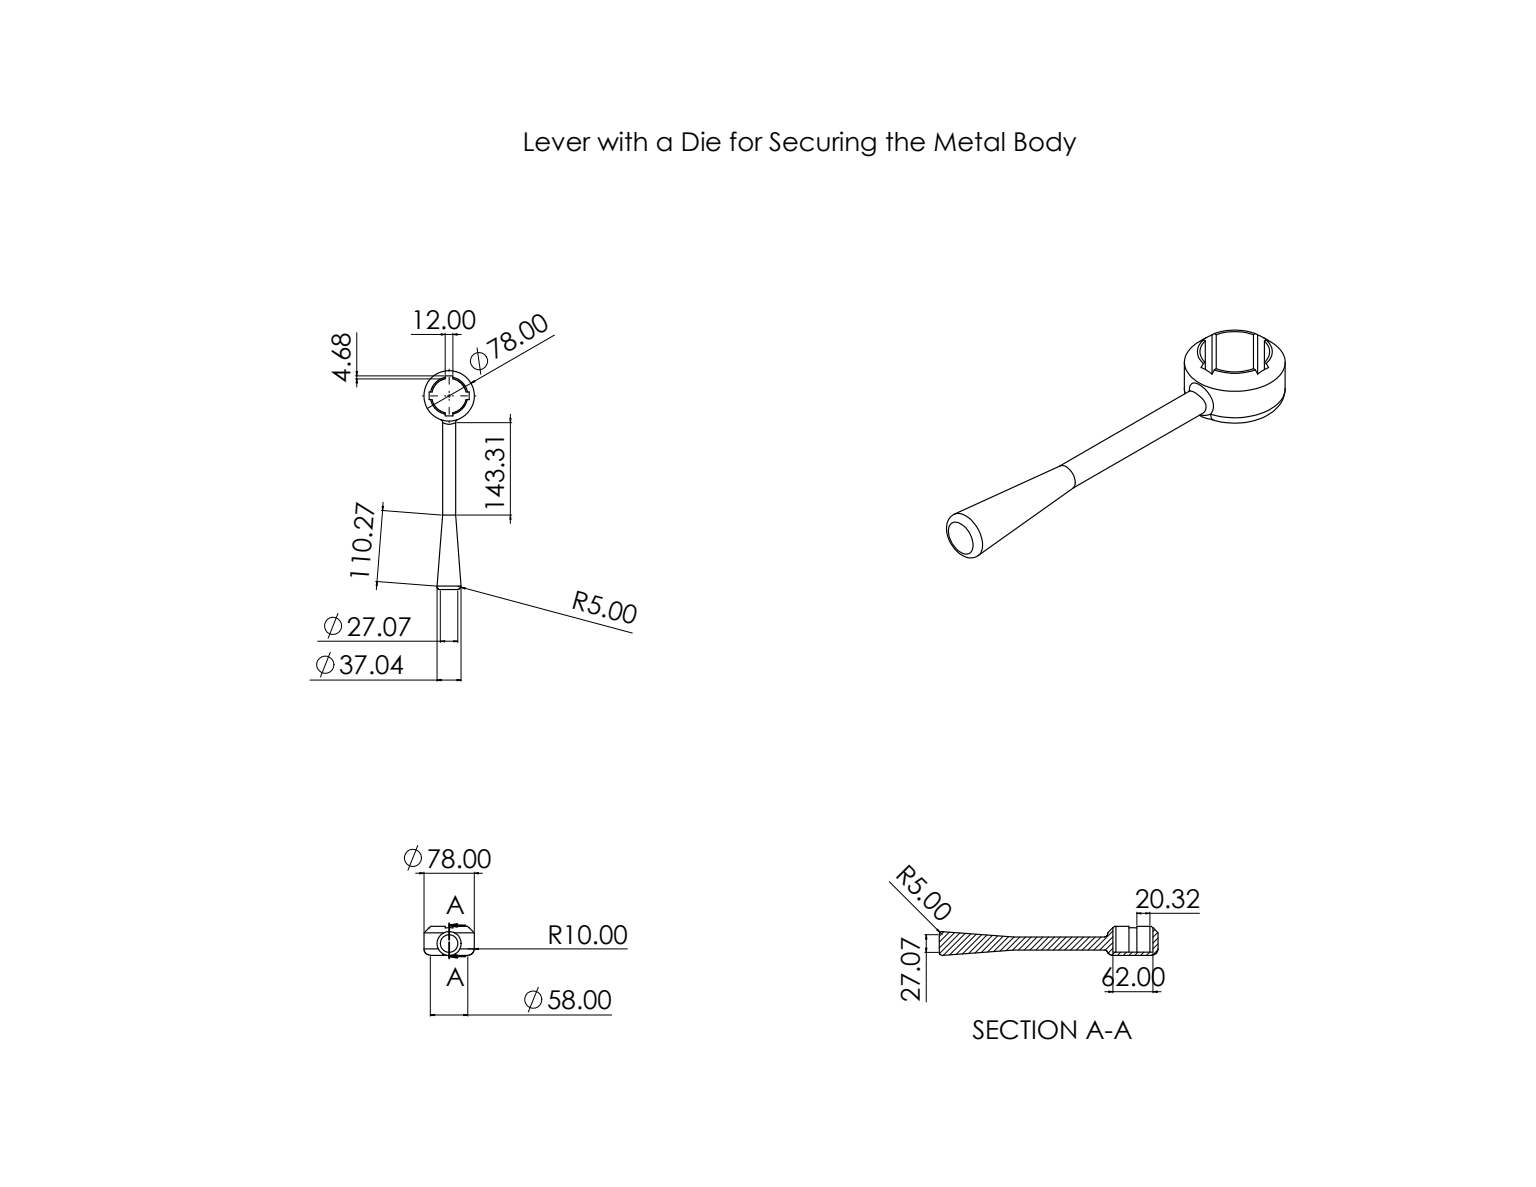
ISO-10303-21;
HEADER;
FILE_DESCRIPTION (('STEP AP214'),
    '1' );
FILE_NAME ('Lever with a Die for Securing the Metal Body.step',
    '2026-10-19T14:05:14',
    ( '' ),
    ( '' ),
    'SwSTEP 2.0',
    'SolidWorks 2025',
    '' );
FILE_SCHEMA (( 'AUTOMOTIVE_DESIGN' ));
ENDSEC;

DATA;
#5=CARTESIAN_POINT ( 'NONE',  ( 3.853297297556091738, -8.887944228554063741, 39.26446342091823993 ) ) ;
#10=CARTESIAN_POINT ( 'NONE',  ( 11.49838106938660509, -4.251877780921969219, 37.26706069643609709 ) ) ;
#13=CARTESIAN_POINT ( 'NONE',  ( 6.000000000000007994, -10.00000000000000533, 31.00000000000000711 ) ) ;
#14=CARTESIAN_POINT ( 'NONE',  ( 6.000000000000007994, 28.28385863652523824, 30.12488991936162108 ) ) ;
#20=CARTESIAN_POINT ( 'NONE',  ( -0.01963426291156584666, -6.705128248126137613, 43.99999014335539016 ) ) ;
#27=PLANE ( 'NONE',  #7404 ) ;
#29=CARTESIAN_POINT ( 'NONE',  ( -0.01628753085184865904, -6.705134819200520901, 38.99999783451422530 ) ) ;
#44=DIRECTION ( 'NONE',  ( -1.000000000000000000, 0.000000000000000000, 0.000000000000000000 ) ) ;
#54=CARTESIAN_POINT ( 'NONE',  ( 4.579605370182076030, -8.646111723837565322, 39.15306555959272572 ) ) ;
#55=CIRCLE ( 'NONE', #3026, 27.00000000000000355 ) ;
#62=CARTESIAN_POINT ( 'NONE',  ( 10.00081333311621989, 3.643253863043277363, 37.85858479645732899 ) ) ;
#67=CARTESIAN_POINT ( 'NONE',  ( -26.32489316217636954, -15.00000000000000000, 6.000000000000009770 ) ) ;
#72=CARTESIAN_POINT ( 'NONE',  ( -9.983292374582678264, 3.962892183205132479, 41.37334990339741125 ) ) ;
#82=CARTESIAN_POINT ( 'NONE',  ( -2.771370799027269349, -6.331017003992445602, 38.93346330084214202 ) ) ;
#93=EDGE_CURVE ( 'NONE', #9341, #7266, #8353, .T. ) ;
#97=CARTESIAN_POINT ( 'NONE',  ( -6.850714361783683870, -15.00000000000000000, 28.25199985127544977 ) ) ;
#112=DIRECTION ( 'NONE',  ( 0.000000000000000000, -1.000000000000000000, 0.000000000000000000 ) ) ;
#113=CARTESIAN_POINT ( 'NONE',  ( 2.825938509006990174, -14.99999999999936762, 36.77312956257851084 ) ) ;
#118=ADVANCED_FACE ( 'NONE', ( #1539 ), #6120, .T. ) ;
#122=CARTESIAN_POINT ( 'NONE',  ( 8.958048712684526294, -1.161593745032227565, 41.89873932196367434 ) ) ;
#131=CARTESIAN_POINT ( 'NONE',  ( -7.290079979600610827, 10.14749281417268811, 42.62097616879101025 ) ) ;
#134=ORIENTED_EDGE ( 'NONE', *, *, #5755, .F. ) ;
#136=ORIENTED_EDGE ( 'NONE', *, *, #3165, .T. ) ;
#157=CYLINDRICAL_SURFACE ( 'NONE', #6340, 39.00000000000002132 ) ;
#161=CARTESIAN_POINT ( 'NONE',  ( 1.729137406965966184, -11.61013223293034713, 38.97104407561932504 ) ) ;
#166=EDGE_CURVE ( 'NONE', #996, #8756, #7398, .T. ) ;
#180=ORIENTED_EDGE ( 'NONE', *, *, #6176, .F. ) ;
#181=CARTESIAN_POINT ( 'NONE',  ( -3.564217818894435563, -6.054132172044422333, 43.67637224480981217 ) ) ;
#182=DIRECTION ( 'NONE',  ( 0.000000000000000000, 0.000000000000000000, -1.000000000000000000 ) ) ;
#193=CARTESIAN_POINT ( 'NONE',  ( 5.031243191487485333, 17.19748707720165370, 38.67840086860066151 ) ) ;
#197=EDGE_CURVE ( 'NONE', #4918, #1409, #1885, .T. ) ;
#202=ORIENTED_EDGE ( 'NONE', *, *, #8489, .F. ) ;
#221=CARTESIAN_POINT ( 'NONE',  ( 0.000000000000000000, 30.00000000000000000, 0.000000000000000000 ) ) ;
#229=ORIENTED_EDGE ( 'NONE', *, *, #4215, .T. ) ;
#244=AXIS2_PLACEMENT_3D ( 'NONE', #7628, #7725, #2222 ) ;
#253=FACE_OUTER_BOUND ( 'NONE', #1428, .T. ) ;
#257=CIRCLE ( 'NONE', #6534, 9.999999999999998224 ) ;
#266=ORIENTED_EDGE ( 'NONE', *, *, #8114, .T. ) ;
#271=CARTESIAN_POINT ( 'NONE',  ( 29.24912810952613640, 29.14236109046821710, 6.000000000000000000 ) ) ;
#282=CARTESIAN_POINT ( 'NONE',  ( -9.999399707319170716, 3.681889571620033497, 37.85894501931166900 ) ) ;
#283=LINE ( 'NONE', #3269, #6859 ) ;
#285=VERTEX_POINT ( 'NONE', #824 ) ;
#292=ADVANCED_FACE ( 'NONE', ( #3127 ), #3178, .T. ) ;
#301=CARTESIAN_POINT ( 'NONE',  ( -5.022008081159694548, 11.94856982034775683, 43.35258044418206680 ) ) ;
#306=ORIENTED_EDGE ( 'NONE', *, *, #6531, .F. ) ;
#322=CARTESIAN_POINT ( 'NONE',  ( -6.860056060574510894, -3.988295739037161614, 42.78128744368499525 ) ) ;
#324=CARTESIAN_POINT ( 'NONE',  ( 3.796404955196288922E-15, 27.99999999999992184, 31.00000000000000711 ) ) ;
#328=DIRECTION ( 'NONE',  ( 8.659560562354889717E-17, -0.7071067811865512365, 0.7071067811865439090 ) ) ;
#332=CARTESIAN_POINT ( 'NONE',  ( 0.000000000000000000, 30.00000000000000000, 0.000000000000000000 ) ) ;
#351=CARTESIAN_POINT ( 'NONE',  ( 0.5362474655584705818, -6.705996766429416667, 39.00014475790622726 ) ) ;
#357=LINE ( 'NONE', #3258, #4214 ) ;
#371=CARTESIAN_POINT ( 'NONE',  ( -9.589511961634933357, 6.242300754483544267, 37.96120689204327192 ) ) ;
#386=ADVANCED_FACE ( 'NONE', ( #5330 ), #2920, .T. ) ;
#409=CARTESIAN_POINT ( 'NONE',  ( -5.034526734170375661, -14.99999999999968026, 36.79137236871326877 ) ) ;
#415=AXIS2_PLACEMENT_3D ( 'NONE', #8024, #2135, #528 ) ;
#419=AXIS2_PLACEMENT_3D ( 'NONE', #5362, #8372, #1607 ) ;
#420=CARTESIAN_POINT ( 'NONE',  ( 0.2877257019632035728, 13.29444216721321403, 38.99993006065623291 ) ) ;
#422=DIRECTION ( 'NONE',  ( 0.000000000000000000, 0.000000000000000000, -1.000000000000000000 ) ) ;
#432=CARTESIAN_POINT ( 'NONE',  ( -8.138638753224961775, -2.524951670102972834, 42.27347557256990029 ) ) ;
#434=LINE ( 'NONE', #4865, #3505 ) ;
#442=DIRECTION ( 'NONE',  ( -0.000000000000000000, 1.000000000000000000, -0.000000000000000000 ) ) ;
#443=CARTESIAN_POINT ( 'NONE',  ( 26.32489316217636954, -15.00000000000000000, -6.000000000000006217 ) ) ;
#456=ORIENTED_EDGE ( 'NONE', *, *, #4265, .F. ) ;
#458=CARTESIAN_POINT ( 'NONE',  ( -5.494756711108470526, -15.00000000000000000, 28.77837652729955309 ) ) ;
#462=CARTESIAN_POINT ( 'NONE',  ( 1.388289885975153126, 13.20576465663912735, 38.98465863473316517 ) ) ;
#466=ORIENTED_EDGE ( 'NONE', *, *, #4986, .F. ) ;
#469=B_SPLINE_CURVE_WITH_KNOTS ( 'NONE', 3,
 ( #5765, #5813, #7291, #4243, #5075, #9572, #1227, #2791, #8825, #7945, #8085, #8782, #1175, #6496, #7140, #6403, #7195, #5857, #2003, #1322, #493, #8877, #4342, #6592, #9613, #9430, #5024, #2641 ),
 .UNSPECIFIED., .F., .F.,
 ( 4, 2, 2, 2, 2, 2, 2, 2, 2, 2, 2, 2, 2, 4 ),
 ( 0.01587631186740470074, 0.01686737684520415656, 0.01785844182300361585, 0.01984057177860253096, 0.02083163675640198678, 0.02182270173420144607, 0.02281376671200090189, 0.02380483168980036118, 0.02578696164539927629, 0.02677802662319873211, 0.02776909160099819140, 0.02975122155659710305, 0.03074228653439655887, 0.03173335151219601469 ),
 .UNSPECIFIED. ) ;
#474=CARTESIAN_POINT ( 'NONE',  ( -0.4121298502407076403, 18.29573530757822653, 39.00026676411541615 ) ) ;
#483=FACE_OUTER_BOUND ( 'NONE', #5558, .T. ) ;
#484=CARTESIAN_POINT ( 'NONE',  ( 10.76768976630624763, 12.19644567871079488, 37.49298203710821298 ) ) ;
#486=CARTESIAN_POINT ( 'NONE',  ( -5.999999999999998224, -15.00000000000000000, 31.00000000000000711 ) ) ;
#487=CIRCLE ( 'NONE', #5977, 29.00000000000001776 ) ;
#493=CARTESIAN_POINT ( 'NONE',  ( 4.177119896625375972, 12.38650817078062083, 43.55397297161687220 ) ) ;
#497=CARTESIAN_POINT ( 'NONE',  ( 7.710389085651311980, -7.163490336350744059, 38.44899322361341376 ) ) ;
#503=CARTESIAN_POINT ( 'NONE',  ( -2.609644126788640328, -9.208034112191455733, 39.41000430683886435 ) ) ;
#505=CARTESIAN_POINT ( 'NONE',  ( 6.000000000000001776, 27.42469319230600533, -31.00000000000000711 ) ) ;
#507=CARTESIAN_POINT ( 'NONE',  ( 8.142856695446859305, 15.19239146806992125, 38.14742590042245496 ) ) ;
#513=ORIENTED_EDGE ( 'NONE', *, *, #7286, .F. ) ;
#519=B_SPLINE_CURVE_WITH_KNOTS ( 'NONE', 3,
 ( #6161, #3804, #5389, #1530 ),
 .UNSPECIFIED., .F., .F.,
 ( 4, 4 ),
 ( 9.813077866773594792E-18, 0.003679109433542027217 ),
 .UNSPECIFIED. ) ;
#520=CARTESIAN_POINT ( 'NONE',  ( -5.000088184532109459, 11.96127634219708291, 43.35829465038302999 ) ) ;
#521=EDGE_CURVE ( 'NONE', #3666, #5938, #5175, .T. ) ;
#528=DIRECTION ( 'NONE',  ( 0.000000000000000000, 0.000000000000000000, -1.000000000000000000 ) ) ;
#536=CARTESIAN_POINT ( 'NONE',  ( 8.924601364836032502, 14.41850173042159433, 37.96585739592215702 ) ) ;
#539=CARTESIAN_POINT ( 'NONE',  ( -28.37252191822215863, 30.00000000000000000, 6.000000000000009770 ) ) ;
#541=ADVANCED_FACE ( 'NONE', ( #6547 ), #5764, .T. ) ;
#546=EDGE_LOOP ( 'NONE', ( #4268, #589, #822, #6096, #5200 ) ) ;
#548=LINE ( 'NONE', #5078, #2613 ) ;
#549=DIRECTION ( 'NONE',  ( 0.000000000000000000, -1.000000000000000000, 0.000000000000000000 ) ) ;
#550=CARTESIAN_POINT ( 'NONE',  ( 11.07761026121386294, -5.000000000000018652, 37.39366993089406321 ) ) ;
#556=CARTESIAN_POINT ( 'NONE',  ( 0.1989820186609699559, -14.99999999999991829, 36.76396650344398864 ) ) ;
#560=CARTESIAN_POINT ( 'NONE',  ( 4.161522685292555757, 12.39367310823792145, 43.55734157098922310 ) ) ;
#569=AXIS2_PLACEMENT_3D ( 'NONE', #6747, #8347, #8246 ) ;
#570=CARTESIAN_POINT ( 'NONE',  ( -5.877770207244633838, 16.75843190384220804, 38.55650392976755114 ) ) ;
#576=CONICAL_SURFACE ( 'NONE', #6079, 10.00000000000001421, 0.07734202994352787353 ) ;
#577=VERTEX_POINT ( 'NONE', #6443 ) ;
#581=CARTESIAN_POINT ( 'NONE',  ( 0.000000000000000000, 30.00000000000000000, 0.000000000000000000 ) ) ;
#587=VECTOR ( 'NONE', #9325, 1000.000000000000000 ) ;
#589=ORIENTED_EDGE ( 'NONE', *, *, #6961, .T. ) ;
#600=FACE_OUTER_BOUND ( 'NONE', #8417, .T. ) ;
#605=CARTESIAN_POINT ( 'NONE',  ( 11.29943480391912480, 11.21459584331072712, 37.32807029000129972 ) ) ;
#610=LINE ( 'NONE', #1297, #1967 ) ;
#614=CARTESIAN_POINT ( 'NONE',  ( -10.79121869663144651, 12.07057269213421691, 37.47816149638868666 ) ) ;
#625=ORIENTED_EDGE ( 'NONE', *, *, #1724, .T. ) ;
#629=PLANE ( 'NONE',  #8412 ) ;
#640=ORIENTED_EDGE ( 'NONE', *, *, #8427, .F. ) ;
#641=CARTESIAN_POINT ( 'NONE',  ( 31.00000000000000711, -10.00000000000000533, -6.000000000000006217 ) ) ;
#642=CARTESIAN_POINT ( 'NONE',  ( 6.848559158582876449, -14.99999999999999822, 28.25275382443572525 ) ) ;
#644=AXIS2_PLACEMENT_3D ( 'NONE', #4878, #3192, #6296 ) ;
#646=EDGE_CURVE ( 'NONE', #1381, #4052, #9276, .T. ) ;
#650=CARTESIAN_POINT ( 'NONE',  ( 9.569793796949216613, 0.3522634836077675469, 37.96578825203867780 ) ) ;
#658=ORIENTED_EDGE ( 'NONE', *, *, #8055, .F. ) ;
#661=CARTESIAN_POINT ( 'NONE',  ( -6.789484220152367300, 10.67953771436871691, 38.52138918282914659 ) ) ;
#669=DIRECTION ( 'NONE',  ( 1.000000000000000000, 0.000000000000000000, 0.000000000000000000 ) ) ;
#681=CARTESIAN_POINT ( 'NONE',  ( -31.00000000000001066, 28.00044749928606791, 0.9877776005181286845 ) ) ;
#693=CARTESIAN_POINT ( 'NONE',  ( 3.829830809861694441, -15.00000000000031619, 36.77956184265733697 ) ) ;
#705=ADVANCED_FACE ( 'NONE', ( #7547 ), #776, .F. ) ;
#719=AXIS2_PLACEMENT_3D ( 'NONE', #3811, #4556, #6908 ) ;
#735=CARTESIAN_POINT ( 'NONE',  ( -6.704071815732007167, 16.26702755093696240, 38.42308545116613061 ) ) ;
#741=CARTESIAN_POINT ( 'NONE',  ( 4.138326062248817827, -15.00000000000031442, 36.78203384243531815 ) ) ;
#743=DIRECTION ( 'NONE',  ( 0.000000000000000000, 0.000000000000000000, 1.000000000000000000 ) ) ;
#750=CARTESIAN_POINT ( 'NONE',  ( 13.27537549950361750, 4.257531348894068479, 36.67105783558309895 ) ) ;
#751=ORIENTED_EDGE ( 'NONE', *, *, #8313, .F. ) ;
#755=CARTESIAN_POINT ( 'NONE',  ( -26.32489316217636954, 30.00000000000000000, 6.000000000000009770 ) ) ;
#756=EDGE_LOOP ( 'NONE', ( #6277, #2707, #2259, #1745, #813, #6889 ) ) ;
#761=EDGE_CURVE ( 'NONE', #1456, #8266, #8388, .T. ) ;
#767=CARTESIAN_POINT ( 'NONE',  ( -28.37252191822216218, 30.00000000000000000, -5.999999999999996447 ) ) ;
#776=PLANE ( 'NONE',  #7111 ) ;
#778=CARTESIAN_POINT ( 'NONE',  ( -2.813731784447083495, -15.00000000000000178, 29.91201187495168412 ) ) ;
#779=CARTESIAN_POINT ( 'NONE',  ( 8.237197373723128990, -15.00000000000000000, 27.80554943579302574 ) ) ;
#789=CARTESIAN_POINT ( 'NONE',  ( 3.173702698177182313, -14.99999999999968736, 36.77512248518149107 ) ) ;
#791=ORIENTED_EDGE ( 'NONE', *, *, #3597, .T. ) ;
#797=CARTESIAN_POINT ( 'NONE',  ( 9.984897811736454187, 3.936638391489574396, 41.37247550685020059 ) ) ;
#800=CARTESIAN_POINT ( 'NONE',  ( 6.000000000000007994, -15.00000000000000000, 31.00000000000000711 ) ) ;
#805=CARTESIAN_POINT ( 'NONE',  ( 1.221566888952841201E-22, 27.99999999999992184, -31.00000000000000711 ) ) ;
#808=CARTESIAN_POINT ( 'NONE',  ( -7.945459518470957327, -2.812008134636945655, 42.35892031214973485 ) ) ;
#811=ORIENTED_EDGE ( 'NONE', *, *, #6176, .T. ) ;
#813=ORIENTED_EDGE ( 'NONE', *, *, #5473, .F. ) ;
#814=UNCERTAINTY_MEASURE_WITH_UNIT (LENGTH_MEASURE( 1.000000000000000082E-05 ), #3122, 'distance_accuracy_value', 'NONE');
#817=CARTESIAN_POINT ( 'NONE',  ( -2.621723037464307460, -6.360998902849781089, 43.82648660254912443 ) ) ;
#822=ORIENTED_EDGE ( 'NONE', *, *, #1375, .F. ) ;
#824=CARTESIAN_POINT ( 'NONE',  ( -5.999999999999998224, -10.00000000000000533, 26.32489316217636954 ) ) ;
#825=EDGE_CURVE ( 'NONE', #7758, #8266, #9312, .T. ) ;
#843=CARTESIAN_POINT ( 'NONE',  ( 0.8530757223511000742, -15.00000000000015987, 36.76494129545336875 ) ) ;
#848=DIRECTION ( 'NONE',  ( 1.000000000000000000, 0.000000000000000000, 0.000000000000000000 ) ) ;
#851=CARTESIAN_POINT ( 'NONE',  ( 8.889207912806641687, -1.327353063715156933, 38.12328956942888425 ) ) ;
#855=DIRECTION ( 'NONE',  ( 1.000000000000000000, 0.000000000000000000, 0.000000000000000000 ) ) ;
#859=CARTESIAN_POINT ( 'NONE',  ( -9.866174171641793222, 4.958453368138042272, 41.43661138559432544 ) ) ;
#867=CARTESIAN_POINT ( 'NONE',  ( -3.062418613096201447, -11.31009261275296218, 38.88193483011423268 ) ) ;
#868=EDGE_CURVE ( 'NONE', #577, #2358, #6977, .T. ) ;
#874=VERTEX_POINT ( 'NONE', #8631 ) ;
#875=CARTESIAN_POINT ( 'NONE',  ( 3.796404955196288922E-15, 27.99999999999992184, 31.00000000000000711 ) ) ;
#888=CIRCLE ( 'NONE', #8608, 27.00000000000000355 ) ;
#897=DIRECTION ( 'NONE',  ( -0.000000000000000000, 1.000000000000000000, -0.000000000000000000 ) ) ;
#898=ORIENTED_EDGE ( 'NONE', *, *, #5824, .F. ) ;
#902=CARTESIAN_POINT ( 'NONE',  ( 6.828744152548106960, -4.017693012958108767, 42.79257513738735241 ) ) ;
#913=CARTESIAN_POINT ( 'NONE',  ( -5.512087641164731266, -8.278301759323600351, 38.98172623838953399 ) ) ;
#915=VERTEX_POINT ( 'NONE', #7983 ) ;
#916=EDGE_CURVE ( 'NONE', #5506, #2973, #8028, .T. ) ;
#917=CARTESIAN_POINT ( 'NONE',  ( -3.052805839235613661, -6.247915692633487339, 38.91814572147156781 ) ) ;
#925=CARTESIAN_POINT ( 'NONE',  ( 28.37252191822216218, 30.00000000000000000, 6.000000000000000000 ) ) ;
#926=CARTESIAN_POINT ( 'NONE',  ( 2.603483962722058287, 18.02285644508602402, 38.91836598778383660 ) ) ;
#932=EDGE_LOOP ( 'NONE', ( #6935, #6466, #9602, #8022, #6551 ) ) ;
#941=EDGE_LOOP ( 'NONE', ( #8806, #3621, #640, #6708, #7358 ) ) ;
#943=CARTESIAN_POINT ( 'NONE',  ( 0.8597079678303534145, -11.70708081913769050, 39.00058418212047684 ) ) ;
#954=CARTESIAN_POINT ( 'NONE',  ( -9.934621505046441925, 1.974978613517290427, 41.40018739529156022 ) ) ;
#960=VERTEX_POINT ( 'NONE', #7329 ) ;
#961=CARTESIAN_POINT ( 'NONE',  ( -6.703682056317219029, -9.695813972231860589, 38.42653128846041000 ) ) ;
#968=ORIENTED_EDGE ( 'NONE', *, *, #8427, .T. ) ;
#975=CARTESIAN_POINT ( 'NONE',  ( 0.7189834692050188769, -15.00000000000000000, 30.52844133725295706 ) ) ;
#985=CARTESIAN_POINT ( 'NONE',  ( -13.53485947486097984, 3.294852476641296768, 295.0000000000000000 ) ) ;
#989=CARTESIAN_POINT ( 'NONE',  ( 1.902041552336364516, -6.533359847113549890, 38.97006628291147479 ) ) ;
#992=CIRCLE ( 'NONE', #6347, 27.00000000000000355 ) ;
#993=ORIENTED_EDGE ( 'NONE', *, *, #2276, .F. ) ;
#996=VERTEX_POINT ( 'NONE', #5804 ) ;
#1009=CARTESIAN_POINT ( 'NONE',  ( -8.134414903913882000, -8.580173454344276252, 38.14378512097410123 ) ) ;
#1020=CARTESIAN_POINT ( 'NONE',  ( 10.00000000000001599, 3.294852476638864491, 41.36423575989288537 ) ) ;
#1034=CARTESIAN_POINT ( 'NONE',  ( -6.109228642973866918, 11.23818579777762139, 43.04298740074260365 ) ) ;
#1039=CARTESIAN_POINT ( 'NONE',  ( 7.734310478464688110, -8.915650141914058580, 38.22714239730741070 ) ) ;
#1041=AXIS2_PLACEMENT_3D ( 'NONE', #3721, #2820, #5974 ) ;
#1057=CARTESIAN_POINT ( 'NONE',  ( -10.00116243144523231, 2.568931457825094355, 37.85849583813012487 ) ) ;
#1064=DIRECTION ( 'NONE',  ( 0.000000000000000000, 0.000000000000000000, -1.000000000000000000 ) ) ;
#1073=EDGE_CURVE ( 'NONE', #8597, #6324, #9168, .T. ) ;
#1078=ORIENTED_EDGE ( 'NONE', *, *, #6544, .F. ) ;
#1084=LINE ( 'NONE', #8592, #6385 ) ;
#1085=CARTESIAN_POINT ( 'NONE',  ( 3.212268717265503337, -6.180893100220475667, 43.73795460093941756 ) ) ;
#1089=VERTEX_POINT ( 'NONE', #2538 ) ;
#1092=ORIENTED_EDGE ( 'NONE', *, *, #6366, .T. ) ;
#1099=ORIENTED_EDGE ( 'NONE', *, *, #6311, .T. ) ;
#1103=AXIS2_PLACEMENT_3D ( 'NONE', #3382, #9423, #7133 ) ;
#1106=CARTESIAN_POINT ( 'NONE',  ( -12.95718999772756952, -0.1032853105602432597, 36.78477091561097723 ) ) ;
#1113=ORIENTED_EDGE ( 'NONE', *, *, #9629, .F. ) ;
#1114=CARTESIAN_POINT ( 'NONE',  ( 13.53485947486097984, 3.294852476641298544, 300.0000000000000000 ) ) ;
#1116=EDGE_LOOP ( 'NONE', ( #4082, #7773, #9193 ) ) ;
#1119=DIRECTION ( 'NONE',  ( -0.000000000000000000, 1.000000000000000000, -0.000000000000000000 ) ) ;
#1141=ORIENTED_EDGE ( 'NONE', *, *, #4794, .F. ) ;
#1147=DIRECTION ( 'NONE',  ( -0.000000000000000000, 1.000000000000000000, -0.000000000000000000 ) ) ;
#1155=ORIENTED_EDGE ( 'NONE', *, *, #3946, .F. ) ;
#1156=ORIENTED_EDGE ( 'NONE', *, *, #6662, .T. ) ;
#1157=CARTESIAN_POINT ( 'NONE',  ( -9.363418156690336502, -0.2310869320007213068, 41.69859845502092099 ) ) ;
#1167=CARTESIAN_POINT ( 'NONE',  ( 0.000000000000000000, -15.00000000000000000, 0.000000000000000000 ) ) ;
#1168=CARTESIAN_POINT ( 'NONE',  ( 11.39612023638420091, -4.438368553505347869, 37.29814521415754314 ) ) ;
#1171=ADVANCED_FACE ( 'NONE', ( #3655 ), #2901, .T. ) ;
#1175=CARTESIAN_POINT ( 'NONE',  ( 7.933835403919273332, 9.390567006709300557, 42.36121793582603345 ) ) ;
#1179=CARTESIAN_POINT ( 'NONE',  ( -9.168699364306950983, 14.24186408291268435, 37.91585989658146616 ) ) ;
#1180=EDGE_CURVE ( 'NONE', #5073, #3751, #2510, .T. ) ;
#1192=CARTESIAN_POINT ( 'NONE',  ( -5.838309802342690702, -8.139381478159863903, 38.91646265135313598 ) ) ;
#1201=CARTESIAN_POINT ( 'NONE',  ( 10.56568760240365457, 12.41321854688487214, 37.54259628649076319 ) ) ;
#1203=VERTEX_POINT ( 'NONE', #2536 ) ;
#1208=EDGE_LOOP ( 'NONE', ( #6379, #6956, #7718, #4930, #229 ) ) ;
#1210=CARTESIAN_POINT ( 'NONE',  ( -9.937482190456421449, 1.998597242238694838, 41.39862281978090408 ) ) ;
#1220=DIRECTION ( 'NONE',  ( 0.000000000000000000, -0.000000000000000000, -1.000000000000000000 ) ) ;
#1221=CARTESIAN_POINT ( 'NONE',  ( 12.17954565146988699, 9.319135634659431844, 37.04959301261877869 ) ) ;
#1227=CARTESIAN_POINT ( 'NONE',  ( 9.479273386569138538, 6.546693577225376259, 41.64111890186204334 ) ) ;
#1232=CARTESIAN_POINT ( 'NONE',  ( 1.020767103194353487, -9.471900692527622567, 39.52815712443386076 ) ) ;
#1240=CARTESIAN_POINT ( 'NONE',  ( -0.8899638032320900116, -15.00000000000000000, 36.76490800571937712 ) ) ;
#1242=ORIENTED_EDGE ( 'NONE', *, *, #9562, .F. ) ;
#1243=DIRECTION ( 'NONE',  ( -1.000000000000000000, -8.673617379884034239E-17, 0.000000000000000000 ) ) ;
#1245=CARTESIAN_POINT ( 'NONE',  ( 1.332947368826647772, 13.21112352634868792, 43.95731769652755361 ) ) ;
#1255=CARTESIAN_POINT ( 'NONE',  ( -3.222268259786776667, 12.78388326438595257, 43.74320717588041418 ) ) ;
#1257=CARTESIAN_POINT ( 'NONE',  ( 4.776122516674679455E-15, -4.999999999999997335, -39.00000000000002132 ) ) ;
#1258=CARTESIAN_POINT ( 'NONE',  ( -5.999999999999998224, 30.00000000000000000, 28.37252191822216218 ) ) ;
#1262=LINE ( 'NONE', #9502, #4913 ) ;
#1266=CARTESIAN_POINT ( 'NONE',  ( 9.573718945232185362, 13.70885271580617371, 37.80730753525386945 ) ) ;
#1268=CARTESIAN_POINT ( 'NONE',  ( 0.000000000000000000, 3.294852476641296768, 184.6745183374407020 ) ) ;
#1273=DIRECTION ( 'NONE',  ( -1.000000000000000000, 0.000000000000000000, 0.000000000000000000 ) ) ;
#1287=CARTESIAN_POINT ( 'NONE',  ( -1.713217124479214482, -14.99999999999999822, 36.76766103293256549 ) ) ;
#1288=EDGE_CURVE ( 'NONE', #6115, #7606, #1262, .T. ) ;
#1292=CARTESIAN_POINT ( 'NONE',  ( 7.946841957352148711, 9.373763190100603993, 42.35574965673851722 ) ) ;
#1297=CARTESIAN_POINT ( 'NONE',  ( 10.00000000000001599, 3.294852476641296768, 300.0000000000000000 ) ) ;
#1301=CARTESIAN_POINT ( 'NONE',  ( -7.505748137593764469, 9.946373970317027968, 38.40043516335172313 ) ) ;
#1315=CARTESIAN_POINT ( 'NONE',  ( 12.79072861028647168, -0.8504798754438103181, 36.84338291468104387 ) ) ;
#1322=CARTESIAN_POINT ( 'NONE',  ( 4.473343921463067474, 12.24450654772725855, 43.48755112989530147 ) ) ;
#1331=CARTESIAN_POINT ( 'NONE',  ( -0.7293704418356496966, -15.00000000000000000, 30.52676338768143083 ) ) ;
#1338=CARTESIAN_POINT ( 'NONE',  ( 7.755618280887227378, 9.651396785365637498, 38.35455593997478729 ) ) ;
#1345=VERTEX_POINT ( 'NONE', #4379 ) ;
#1349=CARTESIAN_POINT ( 'NONE',  ( -5.501707247662611877, 11.70083553198481319, 38.70428226897013957 ) ) ;
#1360=EDGE_CURVE ( 'NONE', #3751, #9075, #4593, .T. ) ;
#1373=DIRECTION ( 'NONE',  ( -1.000000000000000000, 0.000000000000000000, 0.000000000000000000 ) ) ;
#1375=EDGE_CURVE ( 'NONE', #3666, #996, #2781, .T. ) ;
#1379=CARTESIAN_POINT ( 'NONE',  ( 0.02451486836956002016, 18.29482697815588566, 38.99999229514322252 ) ) ;
#1381=VERTEX_POINT ( 'NONE', #2170 ) ;
#1387=CARTESIAN_POINT ( 'NONE',  ( 8.139368704184242631, 9.113401726372073242, 42.27313584737455443 ) ) ;
#1396=CARTESIAN_POINT ( 'NONE',  ( -10.53299942811007917, 12.46136332956525905, 37.55180211538850443 ) ) ;
#1409=VERTEX_POINT ( 'NONE', #8914 ) ;
#1417=CARTESIAN_POINT ( 'NONE',  ( -31.00000000000000711, 27.42469319230601243, -5.999999999999996447 ) ) ;
#1418=EDGE_CURVE ( 'NONE', #1760, #8960, #8774, .T. ) ;
#1420=AXIS2_PLACEMENT_3D ( 'NONE', #332, #9364, #7235 ) ;
#1422=CARTESIAN_POINT ( 'NONE',  ( 31.00000000000001066, 28.00044749928606791, -0.9877776005181261310 ) ) ;
#1424=DIRECTION ( 'NONE',  ( 0.000000000000000000, -1.000000000000000000, 0.000000000000000000 ) ) ;
#1425=EDGE_LOOP ( 'NONE', ( #811, #2910, #8328, #5890, #5870 ) ) ;
#1427=CARTESIAN_POINT ( 'NONE',  ( 0.7189834697752452985, -15.00000000000000000, 30.52844133987663611 ) ) ;
#1428=EDGE_LOOP ( 'NONE', ( #3995, #9372, #9203, #5540, #5218, #9162, #751, #1113, #6522, #9139, #8470, #7506 ) ) ;
#1434=CARTESIAN_POINT ( 'NONE',  ( 9.994974281626689105, -6.644405053951256690, 37.70273452987021301 ) ) ;
#1442=CARTESIAN_POINT ( 'NONE',  ( -0.6382276400259029314, 13.27990715202770566, 43.99233959860035981 ) ) ;
#1446=TOROIDAL_SURFACE ( 'NONE', #4772, 13.53485947486097984, 5.000000000000000000 ) ;
#1448=CARTESIAN_POINT ( 'NONE',  ( -11.07761026121387538, -4.999999999999996447, 37.39366993089406321 ) ) ;
#1456=VERTEX_POINT ( 'NONE', #4622 ) ;
#1460=CARTESIAN_POINT ( 'NONE',  ( 28.37252191822215863, 30.00000000000000000, -6.000000000000006217 ) ) ;
#1464=VECTOR ( 'NONE', #9037, 1000.000000000000000 ) ;
#1465=CARTESIAN_POINT ( 'NONE',  ( 31.00000000000001066, 27.61361909880193011, -5.005767756411733771 ) ) ;
#1477=CARTESIAN_POINT ( 'NONE',  ( 12.57968859814066853, -1.585441976847065115, 36.91571372862268419 ) ) ;
#1484=ORIENTED_EDGE ( 'NONE', *, *, #8532, .F. ) ;
#1505=CARTESIAN_POINT ( 'NONE',  ( -0.02206928620401079830, -9.470079073673241865, 39.52734620791224529 ) ) ;
#1517=CARTESIAN_POINT ( 'NONE',  ( -1.435128562106514627, -15.00000000000000000, 30.37910620731054934 ) ) ;
#1518=DIRECTION ( 'NONE',  ( -0.000000000000000000, 1.000000000000000000, -0.000000000000000000 ) ) ;
#1520=DIRECTION ( 'NONE',  ( 0.000000000000000000, 0.000000000000000000, -1.000000000000000000 ) ) ;
#1526=CARTESIAN_POINT ( 'NONE',  ( 3.475328499451850295, -15.00000000000000000, 29.62685825611925949 ) ) ;
#1530=CARTESIAN_POINT ( 'NONE',  ( -6.000000000000005329, 30.00000000000000000, -28.37252191822215863 ) ) ;
#1532=CARTESIAN_POINT ( 'NONE',  ( 8.973048768580328627, 7.721000296853482325, 41.89150708015632318 ) ) ;
#1537=CARTESIAN_POINT ( 'NONE',  ( -26.32489316217636954, 30.00000000000000000, -5.999999999999995559 ) ) ;
#1539=FACE_OUTER_BOUND ( 'NONE', #941, .T. ) ;
#1542=DIRECTION ( 'NONE',  ( 1.000000000000000000, 0.000000000000000000, 0.000000000000000000 ) ) ;
#1545=CARTESIAN_POINT ( 'NONE',  ( -9.476145798193694958, 6.556557297351624847, 41.64275554677251989 ) ) ;
#1547=CARTESIAN_POINT ( 'NONE',  ( -1.350099534931790579, -6.635463807265971070, 43.96408345250505079 ) ) ;
#1554=ORIENTED_EDGE ( 'NONE', *, *, #7273, .T. ) ;
#1557=CARTESIAN_POINT ( 'NONE',  ( -1.781073977724889623, -11.60243029782703594, 38.96871605616770751 ) ) ;
#1575=DIRECTION ( 'NONE',  ( 1.000000000000000000, 0.000000000000000000, 0.000000000000000000 ) ) ;
#1580=CARTESIAN_POINT ( 'NONE',  ( 4.481683998297255833, -15.00000000000000000, 29.20001163310385905 ) ) ;
#1586=CARTESIAN_POINT ( 'NONE',  ( 13.12535147532733504, 5.736527869694620918, 36.72510388254905678 ) ) ;
#1596=CARTESIAN_POINT ( 'NONE',  ( -2.000890828875744099, 27.95155599451149442, -31.00000000000001066 ) ) ;
#1602=EDGE_LOOP ( 'NONE', ( #8995, #8351, #1554, #5556 ) ) ;
#1607=DIRECTION ( 'NONE',  ( -1.000000000000000000, 0.000000000000000000, 0.000000000000000000 ) ) ;
#1614=CARTESIAN_POINT ( 'NONE',  ( 6.611979057083408939, -4.234811449640147885, 42.87340679459065029 ) ) ;
#1617=LINE ( 'NONE', #3033, #2215 ) ;
#1626=CARTESIAN_POINT ( 'NONE',  ( 8.821391692846543009, -15.00000000000000178, 36.98463040684644909 ) ) ;
#1632=CARTESIAN_POINT ( 'NONE',  ( 8.719889270409380444, -1.642155660953823926, 38.16040262559969420 ) ) ;
#1635=LINE ( 'NONE', #7567, #2917 ) ;
#1647=CARTESIAN_POINT ( 'NONE',  ( -1.109536816265070058, -6.661247609618464516, 38.99263510515930165 ) ) ;
#1657=AXIS2_PLACEMENT_3D ( 'NONE', #3222, #3024, #3978 ) ;
#1659=CARTESIAN_POINT ( 'NONE',  ( 8.955614711045242871, -1.166416508362459137, 41.89990723123212035 ) ) ;
#1661=CARTESIAN_POINT ( 'NONE',  ( 31.00000000000000711, 27.42469319230600533, -6.000000000000006217 ) ) ;
#1662=DIRECTION ( 'NONE',  ( 0.000000000000000000, -0.000000000000000000, -1.000000000000000000 ) ) ;
#1664=CARTESIAN_POINT ( 'NONE',  ( -26.32489316217636954, -10.00000000000000533, 6.000000000000009770 ) ) ;
#1671=CIRCLE ( 'NONE', #7981, 18.51991245392837371 ) ;
#1685=CARTESIAN_POINT ( 'NONE',  ( 3.009843071917527535, -11.32397619240443376, 38.88603724746761969 ) ) ;
#1688=CARTESIAN_POINT ( 'NONE',  ( 10.00000000000001421, 3.294852476641296768, 184.6745183374407020 ) ) ;
#1689=DIRECTION ( 'NONE',  ( -0.000000000000000000, 1.000000000000000000, -0.000000000000000000 ) ) ;
#1718=VERTEX_POINT ( 'NONE', #1537 ) ;
#1719=DIRECTION ( 'NONE',  ( 0.000000000000000000, 0.000000000000000000, -1.000000000000000000 ) ) ;
#1723=DIRECTION ( 'NONE',  ( 0.000000000000000000, 0.000000000000000000, 1.000000000000000000 ) ) ;
#1724=EDGE_CURVE ( 'NONE', #6115, #7120, #1635, .T. ) ;
#1737=VECTOR ( 'NONE', #6997, 1000.000000000000000 ) ;
#1739=CARTESIAN_POINT ( 'NONE',  ( -0.6917606027332897645, -6.703808575055850483, 43.99931531168492427 ) ) ;
#1745=ORIENTED_EDGE ( 'NONE', *, *, #646, .F. ) ;
#1747=CARTESIAN_POINT ( 'NONE',  ( -13.29481821656429652, 3.809926294481188691, 36.66398517656647016 ) ) ;
#1755=DIRECTION ( 'NONE',  ( 0.000000000000000000, 0.000000000000000000, -1.000000000000000000 ) ) ;
#1760=VERTEX_POINT ( 'NONE', #8201 ) ;
#1769=CARTESIAN_POINT ( 'NONE',  ( 5.817259163329850935, -4.845482602429197705, 43.12805808941161700 ) ) ;
#1785=DIRECTION ( 'NONE',  ( -1.000000000000000000, 0.000000000000000000, 0.000000000000000000 ) ) ;
#1792=EDGE_CURVE ( 'NONE', #8477, #9075, #4610, .T. ) ;
#1793=CARTESIAN_POINT ( 'NONE',  ( -13.18364556721897429, 5.298907180833983155, 36.70413758096341184 ) ) ;
#1798=CARTESIAN_POINT ( 'NONE',  ( 0.000000000000000000, -15.00000000000000000, 0.000000000000000000 ) ) ;
#1821=CARTESIAN_POINT ( 'NONE',  ( -0.6444271763597331226, 13.27961199780309798, 43.99218798305987121 ) ) ;
#1826=CARTESIAN_POINT ( 'NONE',  ( -0.01628753085184865904, -6.705134819200520901, 38.99999783451422530 ) ) ;
#1828=VERTEX_POINT ( 'NONE', #13 ) ;
#1831=CARTESIAN_POINT ( 'NONE',  ( 2.000890828875750316, 27.95155599451150152, 31.00000000000001421 ) ) ;
#1836=CARTESIAN_POINT ( 'NONE',  ( 0.000000000000000000, 19.99999999999982236, 39.00000000000002132 ) ) ;
#1845=CARTESIAN_POINT ( 'NONE',  ( -6.066055860285464618, -4.695835677951882836, 38.62830766617436495 ) ) ;
#1856=DIRECTION ( 'NONE',  ( 0.000000000000000000, 0.000000000000000000, 1.000000000000000000 ) ) ;
#1865=CARTESIAN_POINT ( 'NONE',  ( -13.15180771621593792, 5.587517427209601095, 36.71572060651241287 ) ) ;
#1870=ORIENTED_EDGE ( 'NONE', *, *, #3165, .F. ) ;
#1874=DIRECTION ( 'NONE',  ( 1.000000000000000000, 0.000000000000000000, 0.000000000000000000 ) ) ;
#1885=CIRCLE ( 'NONE', #8359, 27.00000000000000355 ) ;
#1887=ORIENTED_EDGE ( 'NONE', *, *, #7554, .F. ) ;
#1888=CARTESIAN_POINT ( 'NONE',  ( -9.211085773935334231, -0.6384518674459094267, 38.05061636510622236 ) ) ;
#1901=CARTESIAN_POINT ( 'NONE',  ( 8.239768008128093513, 15.08660039710901657, 38.12250742654718039 ) ) ;
#1914=CARTESIAN_POINT ( 'NONE',  ( -12.77877500440332170, 7.486973052590117028, 36.84754185667136994 ) ) ;
#1921=CARTESIAN_POINT ( 'NONE',  ( -8.124805145827266983, -15.00000000000000000, 36.91741529765116780 ) ) ;
#1923=VERTEX_POINT ( 'NONE', #8594 ) ;
#1928=CARTESIAN_POINT ( 'NONE',  ( 6.697485916193928190, 16.26204223369385460, 38.42259331311452542 ) ) ;
#1936=CARTESIAN_POINT ( 'NONE',  ( -8.755997409701210543, -1.617811598344234048, 38.15348978656172818 ) ) ;
#1945=CARTESIAN_POINT ( 'NONE',  ( -29.24912810952613640, 29.14236109046821710, -5.999999999999996447 ) ) ;
#1946=CARTESIAN_POINT ( 'NONE',  ( 7.754649722547835466, 15.49890469874339871, 38.22487108103376841 ) ) ;
#1967=VECTOR ( 'NONE', #9594, 1000.000000000000000 ) ;
#1971=CARTESIAN_POINT ( 'NONE',  ( -8.643728504328578310, -6.580413251913810768, 38.16276976896127593 ) ) ;
#1973=CARTESIAN_POINT ( 'NONE',  ( 13.53485947486097984, 3.294852476641298544, 295.0000000000000000 ) ) ;
#1979=CARTESIAN_POINT ( 'NONE',  ( 7.068581912135081247, 16.00861037931602127, 38.35581056696806712 ) ) ;
#1985=EDGE_LOOP ( 'NONE', ( #6670, #9493, #5390, #2665, #2718 ) ) ;
#1987=CARTESIAN_POINT ( 'NONE',  ( -8.768074816142425121, 14.61274975128556264, 38.00682554133690871 ) ) ;
#2003=CARTESIAN_POINT ( 'NONE',  ( 5.048957243282207408, 11.93285829901166295, 43.34552440119345107 ) ) ;
#2010=CYLINDRICAL_SURFACE ( 'NONE', #8911, 27.00000000000000355 ) ;
#2013=CARTESIAN_POINT ( 'NONE',  ( -11.07761026121418091, -4.999999999999992006, 37.39366993089505797 ) ) ;
#2016=ADVANCED_FACE ( 'NONE', ( #9583 ), #2010, .F. ) ;
#2020=CARTESIAN_POINT ( 'NONE',  ( 0.5600451362621369222, 13.28348936595889107, 38.99807195037084995 ) ) ;
#2039=CYLINDRICAL_SURFACE ( 'NONE', #8669, 39.00000000000002132 ) ;
#2047=DIRECTION ( 'NONE',  ( -0.000000000000000000, 0.000000000000000000, -1.000000000000000000 ) ) ;
#2054=LINE ( 'NONE', #5774, #6969 ) ;
#2060=CARTESIAN_POINT ( 'NONE',  ( -8.237197373723452287, -14.99999999999999822, 27.80554943579402405 ) ) ;
#2066=CARTESIAN_POINT ( 'NONE',  ( 6.124541788014690624, 11.22654513750760330, 43.03812152903055477 ) ) ;
#2077=CARTESIAN_POINT ( 'NONE',  ( -8.102752655081463473, 15.22736282390319040, 38.15602848768372723 ) ) ;
#2085=ORIENTED_EDGE ( 'NONE', *, *, #1360, .T. ) ;
#2086=CARTESIAN_POINT ( 'NONE',  ( 6.000000000000001776, 30.00000000000000000, -31.00000000000000711 ) ) ;
#2088=CARTESIAN_POINT ( 'NONE',  ( 0.000000000000000000, 3.294852476641296768, 300.0000000000000000 ) ) ;
#2091=CARTESIAN_POINT ( 'NONE',  ( -5.999999999999998224, -10.00000000000000533, 31.00000000000000711 ) ) ;
#2098=CARTESIAN_POINT ( 'NONE',  ( 6.439978105601112524E-15, 18.29485247664131009, 39.00000000000002132 ) ) ;
#2104=CARTESIAN_POINT ( 'NONE',  ( -2.470322857848779918, -15.00000000000000000, 30.03203418347360909 ) ) ;
#2112=CARTESIAN_POINT ( 'NONE',  ( 5.928038920598607042, 16.73037627209208367, 38.54880476822177116 ) ) ;
#2123=EDGE_LOOP ( 'NONE', ( #8637, #6822, #6319, #1242, #7196 ) ) ;
#2125=CARTESIAN_POINT ( 'NONE',  ( -6.594791314557400419, 10.84011732630675695, 42.87949548222016460 ) ) ;
#2130=EDGE_CURVE ( 'NONE', #3412, #3666, #7250, .T. ) ;
#2135=DIRECTION ( 'NONE',  ( 0.000000000000000000, -1.000000000000000000, 0.000000000000000000 ) ) ;
#2136=ORIENTED_EDGE ( 'NONE', *, *, #9140, .F. ) ;
#2154=CARTESIAN_POINT ( 'NONE',  ( 0.4198266780023428568, -14.99999999999984190, 36.76416815479328903 ) ) ;
#2156=DIRECTION ( 'NONE',  ( -1.224646799147353207E-16, 1.000000000000000000, 0.000000000000000000 ) ) ;
#2157=LINE ( 'NONE', #2954, #6691 ) ;
#2158=CARTESIAN_POINT ( 'NONE',  ( 9.981004741123138402, 4.018542934133168210, 37.86365196549936485 ) ) ;
#2159=ORIENTED_EDGE ( 'NONE', *, *, #8489, .T. ) ;
#2166=CARTESIAN_POINT ( 'NONE',  ( -8.731905042198331302, 8.252142515900809272, 38.15876855944379287 ) ) ;
#2170=CARTESIAN_POINT ( 'NONE',  ( -0.01963426291156584666, -6.705128248126137613, 43.99999014335539016 ) ) ;
#2172=ORIENTED_EDGE ( 'NONE', *, *, #3907, .F. ) ;
#2182=CARTESIAN_POINT ( 'NONE',  ( 0.6536441304786463347, -6.706450183173051194, 44.00066613171647845 ) ) ;
#2186=CARTESIAN_POINT ( 'NONE',  ( 4.007921376381021084, 27.80323177039520033, -31.00000000000000711 ) ) ;
#2188=LINE ( 'NONE', #6792, #4017 ) ;
#2189=CARTESIAN_POINT ( 'NONE',  ( 31.00000000000000355, 27.99909559099847911, 2.017392264862529760 ) ) ;
#2193=FACE_OUTER_BOUND ( 'NONE', #5768, .T. ) ;
#2196=( GEOMETRIC_REPRESENTATION_CONTEXT ( 3 ) GLOBAL_UNCERTAINTY_ASSIGNED_CONTEXT ( ( #3771 ) ) GLOBAL_UNIT_ASSIGNED_CONTEXT ( ( #4528, #4383, #2880 ) ) REPRESENTATION_CONTEXT ( 'NONE', 'WORKASPACE' ) );
#2201=CARTESIAN_POINT ( 'NONE',  ( 9.350174078884196049, -0.2661211825927956576, 41.70529496454247464 ) ) ;
#2211=CARTESIAN_POINT ( 'NONE',  ( -4.149849522310169903, 12.39897866860190767, 43.55983959218083612 ) ) ;
#2215=VECTOR ( 'NONE', #2887, 1000.000000000000000 ) ;
#2220=CARTESIAN_POINT ( 'NONE',  ( 6.000000000000001776, 28.28385863652523824, -30.12488991936162108 ) ) ;
#2222=DIRECTION ( 'NONE',  ( 0.001963426291157480824, 0.9999980724767419948, 0.000000000000000000 ) ) ;
#2223=AXIS2_PLACEMENT_3D ( 'NONE', #5491, #3350, #1723 ) ;
#2234=CARTESIAN_POINT ( 'NONE',  ( -10.00000000000001599, 3.294852476641298100, 300.0000000000000000 ) ) ;
#2243=CARTESIAN_POINT ( 'NONE',  ( 0.000000000000000000, -15.00000000000000000, 0.000000000000000000 ) ) ;
#2246=CARTESIAN_POINT ( 'NONE',  ( 0.4484383372385683519, -15.00000000000000000, 30.56042761519584872 ) ) ;
#2250=CARTESIAN_POINT ( 'NONE',  ( 26.32489316217636954, -15.00000000000000000, 6.000000000000000000 ) ) ;
#2256=CARTESIAN_POINT ( 'NONE',  ( 12.43148144571613223, -2.046608012193396942, 36.96605690027389102 ) ) ;
#2259=ORIENTED_EDGE ( 'NONE', *, *, #2546, .F. ) ;
#2260=CARTESIAN_POINT ( 'NONE',  ( -26.32489316217636954, -15.00000000000000000, 6.000000000000009770 ) ) ;
#2265=DIRECTION ( 'NONE',  ( -0.000000000000000000, -0.000000000000000000, 1.000000000000000000 ) ) ;
#2268=CARTESIAN_POINT ( 'NONE',  ( -1.306712379120655632, 13.21469178175683190, 43.95913021330854065 ) ) ;
#2276=EDGE_CURVE ( 'NONE', #2374, #915, #7159, .T. ) ;
#2280=DIRECTION ( 'NONE',  ( 0.000000000000000000, -1.000000000000000000, 0.000000000000000000 ) ) ;
#2281=CARTESIAN_POINT ( 'NONE',  ( -0.02610464500743471528, -11.70511861050984947, 38.99999126342864741 ) ) ;
#2283=CARTESIAN_POINT ( 'NONE',  ( 5.000171879512024908, -8.491196122513333222, 39.08124479469799439 ) ) ;
#2298=VERTEX_POINT ( 'NONE', #5332 ) ;
#2303=FACE_OUTER_BOUND ( 'NONE', #5668, .T. ) ;
#2306=CARTESIAN_POINT ( 'NONE',  ( 6.332203200428770273, -7.897660556950563127, 38.80169624000574657 ) ) ;
#2310=EDGE_LOOP ( 'NONE', ( #7054, #6754 ) ) ;
#2311=CARTESIAN_POINT ( 'NONE',  ( 9.194894985997349224, -0.6766425519222662999, 38.05435396104630996 ) ) ;
#2314=ADVANCED_FACE ( 'NONE', ( #2303 ), #8291, .T. ) ;
#2322=CARTESIAN_POINT ( 'NONE',  ( -2.620222824297394393, 12.96846514759271152, 43.83512211430772965 ) ) ;
#2323=B_SPLINE_CURVE_WITH_KNOTS ( 'NONE', 3,
 ( #8977, #6686, #9721, #1460 ),
 .UNSPECIFIED., .F., .F.,
 ( 4, 4 ),
 ( 9.813077866773594792E-18, 0.003679109433542027217 ),
 .UNSPECIFIED. ) ;
#2325=CARTESIAN_POINT ( 'NONE',  ( -9.351925007598564932, -0.2614073996901185026, 41.70440666569142252 ) ) ;
#2330=VERTEX_POINT ( 'NONE', #5229 ) ;
#2334=CARTESIAN_POINT ( 'NONE',  ( 6.000000000000007994, 30.00000000000000000, 26.32489316217636954 ) ) ;
#2337=DIRECTION ( 'NONE',  ( -1.000000000000000000, 0.000000000000000000, 0.000000000000000000 ) ) ;
#2341=LINE ( 'NONE', #2234, #8706 ) ;
#2349=AXIS2_PLACEMENT_3D ( 'NONE', #7819, #1785, #7766 ) ;
#2353=CARTESIAN_POINT ( 'NONE',  ( 8.119362783942410289, -15.00000000000000000, 36.91696022903513352 ) ) ;
#2358=VERTEX_POINT ( 'NONE', #3994 ) ;
#2362=DIRECTION ( 'NONE',  ( -0.000000000000000000, 0.000000000000000000, -1.000000000000000000 ) ) ;
#2363=CARTESIAN_POINT ( 'NONE',  ( 6.000000000000007994, 30.00000000000000000, 28.37252191822215863 ) ) ;
#2365=CARTESIAN_POINT ( 'NONE',  ( -0.02206928620401079830, -9.470079073673241865, 39.52734620791224529 ) ) ;
#2366=VECTOR ( 'NONE', #44, 1000.000000000000000 ) ;
#2370=DIRECTION ( 'NONE',  ( 0.000000000000000000, 0.000000000000000000, -1.000000000000000000 ) ) ;
#2374=VERTEX_POINT ( 'NONE', #7793 ) ;
#2377=ORIENTED_EDGE ( 'NONE', *, *, #5999, .T. ) ;
#2383=ADVANCED_FACE ( 'NONE', ( #4787 ), #8533, .F. ) ;
#2389=ORIENTED_EDGE ( 'NONE', *, *, #4010, .F. ) ;
#2398=CIRCLE ( 'NONE', #5866, 5.000000000000004441 ) ;
#2409=CARTESIAN_POINT ( 'NONE',  ( 3.017393985291145331, -6.258907930525880126, 38.92018111626612864 ) ) ;
#2426=CARTESIAN_POINT ( 'NONE',  ( -3.886469093799143071, -5.959786720418388306, 38.86437971944521053 ) ) ;
#2436=ORIENTED_EDGE ( 'NONE', *, *, #2546, .T. ) ;
#2453=DIRECTION ( 'NONE',  ( 0.000000000000000000, 0.000000000000000000, -1.000000000000000000 ) ) ;
#2460=LINE ( 'NONE', #5494, #1737 ) ;
#2464=LINE ( 'NONE', #5498, #2936 ) ;
#2467=CARTESIAN_POINT ( 'NONE',  ( -3.270419483466965982, -6.161042622928358803, 43.72827664804632519 ) ) ;
#2474=CARTESIAN_POINT ( 'NONE',  ( -7.065584702402819772, -3.825344972707461100, 38.47648702749351912 ) ) ;
#2483=CARTESIAN_POINT ( 'NONE',  ( -31.00000000000000711, -10.00000000000000533, 6.000000000000009770 ) ) ;
#2489=DIRECTION ( 'NONE',  ( 0.000000000000000000, -1.000000000000000000, 0.000000000000000000 ) ) ;
#2494=ORIENTED_EDGE ( 'NONE', *, *, #8267, .T. ) ;
#2498=AXIS2_PLACEMENT_3D ( 'NONE', #67, #2362, #5396 ) ;
#2499=CARTESIAN_POINT ( 'NONE',  ( 4.404177573089986808, -5.731393103011397372, 38.82088277608229276 ) ) ;
#2508=CARTESIAN_POINT ( 'NONE',  ( 31.00000000000000711, 27.42469319230601243, 6.000000000000000000 ) ) ;
#2510=LINE ( 'NONE', #4069, #5366 ) ;
#2518=CARTESIAN_POINT ( 'NONE',  ( -9.982669663254970516, 3.970470032139787442, 41.37368756539773074 ) ) ;
#2536=CARTESIAN_POINT ( 'NONE',  ( 28.37252191822215863, 30.00000000000000000, -6.000000000000006217 ) ) ;
#2538=CARTESIAN_POINT ( 'NONE',  ( -13.53485947486097984, 3.294852476641296768, 300.0000000000000000 ) ) ;
#2544=CARTESIAN_POINT ( 'NONE',  ( -9.916130411093226016, 4.630053343978718594, 41.40967485888758404 ) ) ;
#2546=EDGE_CURVE ( 'NONE', #4052, #6324, #469, .T. ) ;
#2550=CARTESIAN_POINT ( 'NONE',  ( 6.030565054738658226, -4.722726170226616560, 38.63317537858744544 ) ) ;
#2571=CARTESIAN_POINT ( 'NONE',  ( -10.01570558914089126, -6.581988155506046212, 37.69304774390490564 ) ) ;
#2575=APPLICATION_CONTEXT ( 'automotive_design' ) ;
#2579=DIRECTION ( 'NONE',  ( 0.000000000000000000, 0.000000000000000000, -1.000000000000000000 ) ) ;
#2583=CARTESIAN_POINT ( 'NONE',  ( 12.93945410785518924, -0.2138153430966752699, 36.79108894230666493 ) ) ;
#2586=FACE_OUTER_BOUND ( 'NONE', #3346, .T. ) ;
#2588=AXIS2_PLACEMENT_3D ( 'NONE', #1268, #5711, #6396 ) ;
#2597=CARTESIAN_POINT ( 'NONE',  ( -6.000000000000005329, -15.00000000000000000, -31.00000000000000711 ) ) ;
#2600=CARTESIAN_POINT ( 'NONE',  ( -13.23256407018424063, 1.700849823644902115, 36.68651977394890196 ) ) ;
#2613=VECTOR ( 'NONE', #3594, 1000.000000000000000 ) ;
#2618=VECTOR ( 'NONE', #1518, 1000.000000000000000 ) ;
#2628=CARTESIAN_POINT ( 'NONE',  ( -12.85843207060513116, 7.233932487497670927, 36.81975545894231061 ) ) ;
#2636=PLANE ( 'NONE',  #2823 ) ;
#2641=CARTESIAN_POINT ( 'NONE',  ( 0.01843853345419280837, 13.29483547765106799, 43.99999130734108377 ) ) ;
#2643=CARTESIAN_POINT ( 'NONE',  ( 0.000000000000000000, 19.99999999999982236, -39.00000000000002132 ) ) ;
#2659=CARTESIAN_POINT ( 'NONE',  ( 0.01843853345419369655, 13.29483547765106977, 43.99999130734107666 ) ) ;
#2665=ORIENTED_EDGE ( 'NONE', *, *, #2977, .T. ) ;
#2669=CARTESIAN_POINT ( 'NONE',  ( -7.944109461005667505, -2.787611319100306240, 42.35690170190217430 ) ) ;
#2676=ORIENTED_EDGE ( 'NONE', *, *, #4215, .F. ) ;
#2704=CARTESIAN_POINT ( 'NONE',  ( 0.01225733702461903260, 18.29484822699931001, 38.99999871588790512 ) ) ;
#2705=CARTESIAN_POINT ( 'NONE',  ( -10.07733521876669336, -14.99999999999807621, 37.15918820280854362 ) ) ;
#2707=ORIENTED_EDGE ( 'NONE', *, *, #1073, .T. ) ;
#2711=CONICAL_SURFACE ( 'NONE', #7777, 39.00000000000002132, 0.7853981633974431720 ) ;
#2712=CARTESIAN_POINT ( 'NONE',  ( 3.604595221023451312, 12.64709689291967187, 38.88259557046998083 ) ) ;
#2718=ORIENTED_EDGE ( 'NONE', *, *, #9262, .T. ) ;
#2720=CARTESIAN_POINT ( 'NONE',  ( 0.02451486836953505749, 18.29482697815588921, 38.99999229514322252 ) ) ;
#2722=DIRECTION ( 'NONE',  ( 1.776356839400250465E-15, 0.000000000000000000, -1.000000000000000000 ) ) ;
#2748=CARTESIAN_POINT ( 'NONE',  ( 0.000000000000000000, 30.00000000000000000, 0.000000000000000000 ) ) ;
#2751=CARTESIAN_POINT ( 'NONE',  ( 10.23650415797109758, -5.544651734979271218, 37.65358413834264439 ) ) ;
#2758=CARTESIAN_POINT ( 'NONE',  ( 0.08302437902281271931, -15.00000000000000000, 30.58222658736175248 ) ) ;
#2759=ORIENTED_EDGE ( 'NONE', *, *, #2130, .F. ) ;
#2766=CARTESIAN_POINT ( 'NONE',  ( 4.330416360834490774, 17.51076624374514523, 38.76727366216590553 ) ) ;
#2771=PRODUCT_DEFINITION_CONTEXT ( 'detailed design', #2575, 'design' ) ;
#2777=CARTESIAN_POINT ( 'NONE',  ( -0.3099780140802378403, 13.29544103063097893, 44.00030096464039531 ) ) ;
#2781=LINE ( 'NONE', #5801, #8763 ) ;
#2785=DIRECTION ( 'NONE',  ( -1.000000000000000000, 0.000000000000000000, 0.000000000000000000 ) ) ;
#2791=CARTESIAN_POINT ( 'NONE',  ( 9.099351244776508807, 7.455330879947340783, 41.82994277301750685 ) ) ;
#2795=CARTESIAN_POINT ( 'NONE',  ( -12.78952641536645984, -0.8552499793260514016, 36.84380182560760630 ) ) ;
#2803=CARTESIAN_POINT ( 'NONE',  ( -6.941591473825946323, -15.00000000000000178, 36.84329602096714495 ) ) ;
#2809=CARTESIAN_POINT ( 'NONE',  ( 3.257065296989332559, 12.77212832130460640, 43.73743695198545112 ) ) ;
#2814=ORIENTED_EDGE ( 'NONE', *, *, #2977, .F. ) ;
#2819=CARTESIAN_POINT ( 'NONE',  ( -4.407734956671747639, 12.30199650488687624, 38.81748064356022354 ) ) ;
#2820=DIRECTION ( 'NONE',  ( -0.000000000000000000, 1.000000000000000000, -0.000000000000000000 ) ) ;
#2823=AXIS2_PLACEMENT_3D ( 'NONE', #581, #9559, #1220 ) ;
#2830=DIRECTION ( 'NONE',  ( 0.000000000000000000, 0.000000000000000000, 1.000000000000000000 ) ) ;
#2840=ORIENTED_EDGE ( 'NONE', *, *, #521, .F. ) ;
#2841=LINE ( 'NONE', #2643, #2878 ) ;
#2842=DIRECTION ( 'NONE',  ( 1.000000000000000000, 0.000000000000000000, 0.000000000000000000 ) ) ;
#2850=CARTESIAN_POINT ( 'NONE',  ( -6.850714362160835513, -15.00000000000000000, 28.25199985226410959 ) ) ;
#2852=EDGE_LOOP ( 'NONE', ( #8155, #2377, #5734, #4966 ) ) ;
#2858=CARTESIAN_POINT ( 'NONE',  ( 1.663275198395546939, 13.16107044704059881, 43.93189623020137446 ) ) ;
#2868=ORIENTED_EDGE ( 'NONE', *, *, #9331, .T. ) ;
#2869=CARTESIAN_POINT ( 'NONE',  ( -6.030734287580929553, 11.33421872313606649, 38.63588227429310251 ) ) ;
#2875=ORIENTED_EDGE ( 'NONE', *, *, #5710, .F. ) ;
#2877=TOROIDAL_SURFACE ( 'NONE', #5723, 29.00000000000001776, 10.00000000000000000 ) ;
#2878=VECTOR ( 'NONE', #8878, 1000.000000000000000 ) ;
#2880=( NAMED_UNIT ( * ) SI_UNIT ( $, .STERADIAN. ) SOLID_ANGLE_UNIT ( ) );
#2884=DIRECTION ( 'NONE',  ( -0.000000000000000000, -1.000000000000000000, -0.000000000000000000 ) ) ;
#2887=DIRECTION ( 'NONE',  ( -0.000000000000000000, 1.000000000000000000, -0.000000000000000000 ) ) ;
#2889=CARTESIAN_POINT ( 'NONE',  ( -1.288876940849657649, 18.24222776313161631, 38.98402153286875205 ) ) ;
#2891=CARTESIAN_POINT ( 'NONE',  ( 31.00000000000000711, 27.42469319230601243, 6.000000000000000000 ) ) ;
#2895=CARTESIAN_POINT ( 'NONE',  ( 0.3577198796026725414, -15.00000000000000178, 30.56861933562558775 ) ) ;
#2900=CARTESIAN_POINT ( 'NONE',  ( 26.32489316217636954, 30.00000000000000000, 6.000000000000000000 ) ) ;
#2901=PLANE ( 'NONE',  #2349 ) ;
#2903=CARTESIAN_POINT ( 'NONE',  ( 9.491487835072193846, 6.511041217878577037, 41.63483005588284414 ) ) ;
#2907=EDGE_LOOP ( 'NONE', ( #4763, #5693, #8433, #791 ) ) ;
#2910=ORIENTED_EDGE ( 'NONE', *, *, #9629, .T. ) ;
#2916=CARTESIAN_POINT ( 'NONE',  ( -7.285584084550976947, 10.15239125381765994, 42.62273125021567921 ) ) ;
#2917=VECTOR ( 'NONE', #8352, 1000.000000000000000 ) ;
#2920=CONICAL_SURFACE ( 'NONE', #4202, 39.00000000000002132, 0.7853981633974431720 ) ;
#2921=CIRCLE ( 'NONE', #419, 18.51991245392837371 ) ;
#2933=PLANE ( 'NONE',  #3137 ) ;
#2936=VECTOR ( 'NONE', #8837, 1000.000000000000000 ) ;
#2944=CARTESIAN_POINT ( 'NONE',  ( -5.012544999578074645, 17.20596322573581105, 38.68080642594335927 ) ) ;
#2946=ORIENTED_EDGE ( 'NONE', *, *, #5705, .T. ) ;
#2951=CARTESIAN_POINT ( 'NONE',  ( 1.338007665914787259, -9.401856577713825658, 39.49693264723424591 ) ) ;
#2954=CARTESIAN_POINT ( 'NONE',  ( -26.32489316217636954, 30.00000000000000000, 6.000000000000009770 ) ) ;
#2957=CARTESIAN_POINT ( 'NONE',  ( 7.517587493874460236, -3.331319210360449201, 42.53641844432376473 ) ) ;
#2959=ORIENTED_EDGE ( 'NONE', *, *, #4249, .F. ) ;
#2966=CARTESIAN_POINT ( 'NONE',  ( -5.302731225069202026, 11.77929979337195654, 43.27702668925476104 ) ) ;
#2970=EDGE_CURVE ( 'NONE', #4052, #9341, #610, .T. ) ;
#2971=ORIENTED_EDGE ( 'NONE', *, *, #5705, .F. ) ;
#2973=VERTEX_POINT ( 'NONE', #3612 ) ;
#2975=CARTESIAN_POINT ( 'NONE',  ( 6.000000000000001776, 30.00000000000000000, -28.37252191822216218 ) ) ;
#2977=EDGE_CURVE ( 'NONE', #4609, #285, #3108, .T. ) ;
#2983=EDGE_CURVE ( 'NONE', #1828, #7231, #8405, .T. ) ;
#2988=CARTESIAN_POINT ( 'NONE',  ( 6.000000000000001776, 27.42469319230600533, -31.00000000000000711 ) ) ;
#2996=CARTESIAN_POINT ( 'NONE',  ( 5.828629696051876863, -14.99999999999999822, 28.64426056422739464 ) ) ;
#2997=EDGE_CURVE ( 'NONE', #6561, #915, #4035, .T. ) ;
#2998=VERTEX_POINT ( 'NONE', #2363 ) ;
#3002=CARTESIAN_POINT ( 'NONE',  ( 8.350939762285211287, -2.249335134881106590, 38.23794203041205719 ) ) ;
#3008=CARTESIAN_POINT ( 'NONE',  ( 6.000000000000007994, 30.00000000000000000, 28.37252191822215863 ) ) ;
#3012=CARTESIAN_POINT ( 'NONE',  ( -4.007938479032604917, 27.75794689997812270, -31.00000000000001066 ) ) ;
#3024=DIRECTION ( 'NONE',  ( -0.000000000000000000, 1.000000000000000000, -0.000000000000000000 ) ) ;
#3026=AXIS2_PLACEMENT_3D ( 'NONE', #221, #4562, #2370 ) ;
#3029=VECTOR ( 'NONE', #7095, 1000.000000000000000 ) ;
#3030=ORIENTED_EDGE ( 'NONE', *, *, #7565, .F. ) ;
#3033=CARTESIAN_POINT ( 'NONE',  ( 0.000000000000000000, -15.00000000000000000, 39.00000000000002132 ) ) ;
#3044=CARTESIAN_POINT ( 'NONE',  ( 1.072424122083380116, -9.427504479632391465, 39.50837534435000720 ) ) ;
#3050=EDGE_CURVE ( 'NONE', #7231, #2998, #6441, .T. ) ;
#3051=CARTESIAN_POINT ( 'NONE',  ( 9.914908413137576204, 1.791417294963860041, 37.88076626776848599 ) ) ;
#3052=VECTOR ( 'NONE', #3380, 1000.000000000000000 ) ;
#3053=ORIENTED_EDGE ( 'NONE', *, *, #3736, .T. ) ;
#3074=CARTESIAN_POINT ( 'NONE',  ( -4.738789600095485888, -10.72862449626830106, 38.71314812621989887 ) ) ;
#3075=DIRECTION ( 'NONE',  ( 0.000000000000000000, -1.000000000000000000, 0.000000000000000000 ) ) ;
#3081=DIRECTION ( 'NONE',  ( -0.000000000000000000, 0.000000000000000000, -1.000000000000000000 ) ) ;
#3086=CARTESIAN_POINT ( 'NONE',  ( -7.537829016256761605, -15.00000000000000178, 28.01273236561391045 ) ) ;
#3092=DIRECTION ( 'NONE',  ( 0.000000000000000000, 0.000000000000000000, -1.000000000000000000 ) ) ;
#3096=CARTESIAN_POINT ( 'NONE',  ( 5.021056721195745531, -14.99999999999936229, 36.79118000870545302 ) ) ;
#3098=ADVANCED_FACE ( 'NONE', ( #6017 ), #3917, .T. ) ;
#3100=CARTESIAN_POINT ( 'NONE',  ( 18.51991245392837371, 3.294852476641296768, 294.6136752714472777 ) ) ;
#3103=CARTESIAN_POINT ( 'NONE',  ( 11.27186822886705642, -4.675031839269720990, 37.33643085324619904 ) ) ;
#3104=B_SPLINE_CURVE_WITH_KNOTS ( 'NONE', 3,
 ( #1417, #4437, #6640, #681, #6937, #4645, #5429, #4784 ),
 .UNSPECIFIED., .F., .F.,
 ( 4, 2, 2, 4 ),
 ( 8.673617379884035472E-19, 0.006005055813302546432, 0.009007583719953818346, 0.01201011162660509113 ),
 .UNSPECIFIED. ) ;
#3105=ORIENTED_EDGE ( 'NONE', *, *, #8964, .F. ) ;
#3108=LINE ( 'NONE', #4509, #9237 ) ;
#3122=( LENGTH_UNIT ( ) NAMED_UNIT ( * ) SI_UNIT ( .MILLI., .METRE. ) );
#3123=CARTESIAN_POINT ( 'NONE',  ( 11.07761026121386294, -5.000000000000018652, 37.39366993089406321 ) ) ;
#3127=FACE_OUTER_BOUND ( 'NONE', #546, .T. ) ;
#3133=FACE_OUTER_BOUND ( 'NONE', #7919, .T. ) ;
#3137=AXIS2_PLACEMENT_3D ( 'NONE', #5983, #2280, #6674 ) ;
#3140=TOROIDAL_SURFACE ( 'NONE', #5204, 13.53485947486097984, 5.000000000000000000 ) ;
#3151=CARTESIAN_POINT ( 'NONE',  ( 1.076825440025126701, -6.664617900633762027, 38.99321102797971861 ) ) ;
#3157=CARTESIAN_POINT ( 'NONE',  ( 6.000000000000007994, 27.42469319230600533, 31.00000000000000711 ) ) ;
#3164=AXIS2_PLACEMENT_3D ( 'NONE', #5067, #7385, #8219 ) ;
#3165=EDGE_CURVE ( 'NONE', #9635, #7666, #257, .T. ) ;
#3178=PLANE ( 'NONE',  #4104 ) ;
#3185=CARTESIAN_POINT ( 'NONE',  ( 5.886704555688092810, 16.74912705918251987, 38.55424405853467817 ) ) ;
#3186=LINE ( 'NONE', #1664, #2366 ) ;
#3192=DIRECTION ( 'NONE',  ( -0.9999981025415526359, 0.001843852981148144709, 0.0006285852992236709872 ) ) ;
#3210=CARTESIAN_POINT ( 'NONE',  ( -10.00000000000117595, 2.631365979993403048, 41.36423575989225299 ) ) ;
#3219=CARTESIAN_POINT ( 'NONE',  ( -9.346405976260257376, -0.3019310421636504649, 38.01899321338081705 ) ) ;
#3222=CARTESIAN_POINT ( 'NONE',  ( 0.000000000000000000, 30.00000000000000000, 0.000000000000000000 ) ) ;
#3226=CARTESIAN_POINT ( 'NONE',  ( -5.999999999999998224, 27.42469319230601243, 31.00000000000000711 ) ) ;
#3229=ORIENTED_EDGE ( 'NONE', *, *, #646, .T. ) ;
#3233=PLANE ( 'NONE',  #9634 ) ;
#3244=( BOUNDED_SURFACE ( )  B_SPLINE_SURFACE ( 3, 2, ( 
 ( #6516, #3462, #2659 ),
 ( #6418, #420, #3420 ),
 ( #9632, #2020, #4364 ),
 ( #5148, #8704, #1245 ),
 ( #4307, #462, #2858 ),
 ( #3507, #6461, #5687 ),
 ( #2766, #9487, #2809 ),
 ( #8053, #2712, #560 ),
 ( #2112, #5788, #9448 ),
 ( #1928, #8800, #5733 ),
 ( #1979, #5873, #8894 ),
 ( #507, #4950, #2066 ),
 ( #6568, #5095, #7367 ),
 ( #8749, #7962, #9590 ),
 ( #5831, #8102, #8156 ),
 ( #1201, #5002, #1292 ),
 ( #3563, #1338, #1387 ),
 ( #605, #9538, #8012 ),
 ( #4406, #4259, #3607 ),
 ( #9045, #5238, #1532 ),
 ( #3755, #6655, #5964 ),
 ( #9678, #3657, #2903 ),
 ( #7415, #5922, #3857 ),
 ( #1586, #4552, #5391 ),
 ( #8250, #5289, #6805 ),
 ( #750, #2158, #797 ),
 ( #7564, #62, #8401 ),
 ( #8303, #5341, #3806 ),
 ( #4607, #3051, #7513 ),
 ( #8349, #7464, #6069 ),
 ( #6116, #650, #9100 ),
 ( #1477, #7611, #4502 ),
 ( #2256, #2311, #2201 ),
 ( #6857, #851, #6749 ),
 ( #6706, #1632, #122 ),
 ( #10, #3002, #6011 ),
 ( #3103, #8948, #3705 ),
 ( #5192, #8199, #9143 ),
 ( #1434, #9734, #2957 ),
 ( #8992, #6163, #902 ),
 ( #5535, #2550, #8646 ),
 ( #5633, #4107, #4655 ),
 ( #1039, #8593, #1769 ),
 ( #7662, #2499, #3913 ),
 ( #9289, #8545, #5441 ),
 ( #9194, #2409, #4058 ),
 ( #8453, #7862, #1085 ),
 ( #3252, #7102, #6904 ),
 ( #1685, #989, #7711 ),
 ( #161, #3151, #4704 ),
 ( #943, #351, #6262 ),
 ( #4798, #1826, #3955 ) ),
 .UNSPECIFIED., .F., .F., .F. ) 
 B_SPLINE_SURFACE_WITH_KNOTS ( ( 4, 2, 2, 2, 2, 2, 2, 2, 2, 2, 2, 2, 2, 2, 2, 2, 2, 2, 2, 2, 2, 2, 2, 2, 2, 4 ),
 ( 3, 3 ),
 ( 0.04726531707896113044, 0.04874235823767866793, 0.05021939939639619849, 0.05317348171383126654, 0.05465052287254880403, 0.05612756403126634153, 0.05908164634870140958, 0.06055868750741894013, 0.06203572866613647763, 0.06351276982485401512, 0.06498981098357155262, 0.06794389330100661373, 0.06942093445972415122, 0.07089797561844168872, 0.07385205793587676371, 0.07532909909459430120, 0.07680614025331183869, 0.07828318141202937619, 0.07976022257074691368, 0.08271430488818197480, 0.08419134604689951229, 0.08566838720561703591, 0.08862246952305211090, 0.09009951068176964839, 0.09157655184048718588, 0.09453063415792226087 ),
 ( 0.000000000000000000, 1.000000000000000000 ),
 .UNSPECIFIED. ) 
 GEOMETRIC_REPRESENTATION_ITEM ( )  RATIONAL_B_SPLINE_SURFACE ( (
 ( 1.000000000000000000, 0.7071071909622603791, 1.000000000000000000),
 ( 1.000000000000000000, 0.7071216684788621532, 1.000000000000000000),
 ( 1.000000000000000000, 0.7075267130853096775, 1.000000000000000000),
 ( 1.000000000000000000, 0.7091156140370702410, 1.000000000000000000),
 ( 1.000000000000000000, 0.7103097360554838646, 1.000000000000000000),
 ( 1.000000000000000000, 0.7149216248805696505, 1.000000000000000000),
 ( 1.000000000000000000, 0.7193697620773539247, 1.000000000000000000),
 ( 1.000000000000000000, 0.7275797806198590623, 1.000000000000000000),
 ( 1.000000000000000000, 0.7305845420014355218, 1.000000000000000000),
 ( 1.000000000000000000, 0.7369677174223107086, 1.000000000000000000),
 ( 1.000000000000000000, 0.7403163103353537222, 1.000000000000000000),
 ( 1.000000000000000000, 0.7506600275792891797, 1.000000000000000000),
 ( 1.000000000000000000, 0.7579512107779988739, 1.000000000000000000),
 ( 1.000000000000000000, 0.7688664121945819607, 1.000000000000000000),
 ( 1.000000000000000000, 0.7724869259326714310, 1.000000000000000000),
 ( 1.000000000000000000, 0.7794781267615982223, 1.000000000000000000),
 ( 1.000000000000000000, 0.7828668203034458983, 1.000000000000000000),
 ( 1.000000000000000000, 0.7893489739652082005, 1.000000000000000000),
 ( 1.000000000000000000, 0.7924426342044915694, 1.000000000000000000),
 ( 1.000000000000000000, 0.7982547573422374976, 1.000000000000000000),
 ( 1.000000000000000000, 0.8009870661436891970, 1.000000000000000000),
 ( 1.000000000000000000, 0.8083787752127222781, 1.000000000000000000),
 ( 1.000000000000000000, 0.8122306866419456428, 1.000000000000000000),
 ( 1.000000000000000000, 0.8161590539804731703, 1.000000000000000000),
 ( 1.000000000000000000, 0.8171599891451262199, 1.000000000000000000),
 ( 1.000000000000000000, 0.8184978691222959402, 1.000000000000000000),
 ( 1.000000000000000000, 0.8188263875099578426, 1.000000000000000000),
 ( 1.000000000000000000, 0.8187846005707258845, 1.000000000000000000),
 ( 1.000000000000000000, 0.8174048505046132007, 1.000000000000000000),
 ( 1.000000000000000000, 0.8133903365045817013, 1.000000000000000000),
 ( 1.000000000000000000, 0.8117167614377021057, 1.000000000000000000),
 ( 1.000000000000000000, 0.8078263697157368473, 1.000000000000000000),
 ( 1.000000000000000000, 0.8056055056598052655, 1.000000000000000000),
 ( 1.000000000000000000, 0.8006760202143063943, 1.000000000000000000),
 ( 1.000000000000000000, 0.7979672363511526312, 1.000000000000000000),
 ( 1.000000000000000000, 0.7921221611992056433, 1.000000000000000000),
 ( 1.000000000000000000, 0.7889678644669387841, 1.000000000000000000),
 ( 1.000000000000000000, 0.7791076940979192456, 1.000000000000000000),
 ( 1.000000000000000000, 0.7720256508000469253, 1.000000000000000000),
 ( 1.000000000000000000, 0.7611892740573897864, 1.000000000000000000),
 ( 1.000000000000000000, 0.7575416872336065977, 1.000000000000000000),
 ( 1.000000000000000000, 0.7502769197745564611, 1.000000000000000000),
 ( 1.000000000000000000, 0.7467060562589890038, 1.000000000000000000),
 ( 1.000000000000000000, 0.7363894265406839557, 1.000000000000000000),
 ( 1.000000000000000000, 0.7300094285789220372, 1.000000000000000000),
 ( 1.000000000000000000, 0.7218273080856705270, 1.000000000000000000),
 ( 1.000000000000000000, 0.7193219373239115866, 1.000000000000000000),
 ( 1.000000000000000000, 0.7149816326288559454, 1.000000000000000000),
 ( 1.000000000000000000, 0.7131353591592815011, 1.000000000000000000),
 ( 1.000000000000000000, 0.7086530176431308226, 1.000000000000000000),
 ( 1.000000000000000000, 0.7070745693947934063, 1.000000000000000000),
 ( 1.000000000000000000, 0.7071072458330266430, 1.000000000000000000) ) ) 
 REPRESENTATION_ITEM ( '' )  SURFACE ( )  );
#3250=CARTESIAN_POINT ( 'NONE',  ( -6.000000000000005329, -10.00000000000000533, -31.00000000000000711 ) ) ;
#3252=CARTESIAN_POINT ( 'NONE',  ( 3.432825031707446684, -11.20495311582498310, 38.85090753550943532 ) ) ;
#3258=CARTESIAN_POINT ( 'NONE',  ( -31.00000000000000711, -10.00000000000000533, -5.999999999999996447 ) ) ;
#3259=ORIENTED_EDGE ( 'NONE', *, *, #4085, .T. ) ;
#3260=CARTESIAN_POINT ( 'NONE',  ( 30.12488991936162464, 28.28385863652524179, 6.000000000000000000 ) ) ;
#3262=ORIENTED_EDGE ( 'NONE', *, *, #6293, .T. ) ;
#3264=VERTEX_POINT ( 'NONE', #7808 ) ;
#3268=CARTESIAN_POINT ( 'NONE',  ( -8.802338400919726524, -7.957579170021067405, 37.99520874873245901 ) ) ;
#3269=CARTESIAN_POINT ( 'NONE',  ( 4.776122516674679455E-15, -15.00000000000000000, -39.00000000000002132 ) ) ;
#3276=DIRECTION ( 'NONE',  ( -0.000000000000000000, -1.000000000000000000, -0.000000000000000000 ) ) ;
#3296=CARTESIAN_POINT ( 'NONE',  ( -7.509415180676684898, 9.906480154215739020, 42.53495263954286543 ) ) ;
#3311=FACE_OUTER_BOUND ( 'NONE', #4822, .T. ) ;
#3312=EDGE_CURVE ( 'NONE', #6269, #8597, #7400, .T. ) ;
#3313=LINE ( 'NONE', #7161, #4979 ) ;
#3323=CARTESIAN_POINT ( 'NONE',  ( -9.915904358114350003, 4.630888946090288449, 41.40979624514990576 ) ) ;
#3330=CARTESIAN_POINT ( 'NONE',  ( 9.348208607970679651, -0.2712915440469981232, 41.70628801877622749 ) ) ;
#3346=EDGE_LOOP ( 'NONE', ( #9107, #5455, #7688, #1092 ) ) ;
#3350=DIRECTION ( 'NONE',  ( -0.000000000000000000, 1.000000000000000000, -0.000000000000000000 ) ) ;
#3358=ORIENTED_EDGE ( 'NONE', *, *, #7818, .F. ) ;
#3365=EDGE_LOOP ( 'NONE', ( #625, #5333, #5634, #7729, #4615 ) ) ;
#3372=CARTESIAN_POINT ( 'NONE',  ( -9.671299335021130261, 5.920905817192278597, 41.54023692788936017 ) ) ;
#3375=AXIS2_PLACEMENT_3D ( 'NONE', #3847, #8340, #1575 ) ;
#3380=DIRECTION ( 'NONE',  ( -0.07726494571055114724, 9.462226845072048778E-18, 0.9970105958134776181 ) ) ;
#3382=CARTESIAN_POINT ( 'NONE',  ( 0.000000000000000000, -15.00000000000000000, 0.000000000000000000 ) ) ;
#3383=CIRCLE ( 'NONE', #244, 5.000000000000000888 ) ;
#3384=CARTESIAN_POINT ( 'NONE',  ( 13.16003951335063782, 1.062643319146125087, 36.71276424047989906 ) ) ;
#3387=CARTESIAN_POINT ( 'NONE',  ( -29.24912810952613640, 29.14236109046821710, 6.000000000000009770 ) ) ;
#3394=AXIS2_PLACEMENT_3D ( 'NONE', #4362, #9631, #9589 ) ;
#3403=B_SPLINE_CURVE_WITH_KNOTS ( 'NONE', 3,
 ( #4483, #9078, #9664, #3687, #6685, #6102, #4640, #5903, #7549, #7490, #975, #5996, #9026, #5268, #8281, #1517, #8931, #778, #4588, #3840, #6835, #97, #3086, #6146 ),
 .UNSPECIFIED., .F., .F.,
 ( 4, 2, 2, 2, 2, 2, 2, 2, 2, 2, 2, 4 ),
 ( 0.000000000000000000, 0.002184979252289450703, 0.004369958504578901407, 0.006554937756868352110, 0.007647427383013077895, 0.008193672196085440354, 0.008739917009157802813, 0.009832406635302527731, 0.01092489626144725265, 0.01310987551373670422, 0.01529485476602615579, 0.01747983401831560563 ),
 .UNSPECIFIED. ) ;
#3404=CYLINDRICAL_SURFACE ( 'NONE', #2223, 27.00000000000000355 ) ;
#3412=VERTEX_POINT ( 'NONE', #641 ) ;
#3420=CARTESIAN_POINT ( 'NONE',  ( 0.3468554216641324128, 13.29422992404367143, 43.99968164972226248 ) ) ;
#3430=CARTESIAN_POINT ( 'NONE',  ( -8.989938151044675863, -1.132833736518202628, 41.88450937582585709 ) ) ;
#3434=FACE_OUTER_BOUND ( 'NONE', #1602, .T. ) ;
#3445=ORIENTED_EDGE ( 'NONE', *, *, #1360, .F. ) ;
#3454=CARTESIAN_POINT ( 'NONE',  ( -3.482215743441875233, -15.00000000000000000, 29.62396259739072946 ) ) ;
#3455=EDGE_CURVE ( 'NONE', #874, #3412, #3850, .T. ) ;
#3462=CARTESIAN_POINT ( 'NONE',  ( 0.01529561594344277208, 13.29484127273988570, 38.99999809024075859 ) ) ;
#3466=ORIENTED_EDGE ( 'NONE', *, *, #8609, .F. ) ;
#3470=CARTESIAN_POINT ( 'NONE',  ( -0.2571447251526570721, 13.29524039329391627, 39.00006612239294412 ) ) ;
#3472=DIRECTION ( 'NONE',  ( -1.000000000000000000, 0.000000000000000000, 0.000000000000000000 ) ) ;
#3483=CARTESIAN_POINT ( 'NONE',  ( 12.20502364804429263, -2.690346678627072663, 37.04198800656732260 ) ) ;
#3495=AXIS2_PLACEMENT_3D ( 'NONE', #8633, #7845, #1662 ) ;
#3500=CARTESIAN_POINT ( 'NONE',  ( -1.119899052094893266, -9.430686232357382792, 39.50984196849405805 ) ) ;
#3504=PLANE ( 'NONE',  #9552 ) ;
#3505=VECTOR ( 'NONE', #3472, 1000.000000000000000 ) ;
#3507=CARTESIAN_POINT ( 'NONE',  ( 3.500479179565848309, 17.79940450863160351, 38.85213755562799065 ) ) ;
#3515=ADVANCED_FACE ( 'NONE', ( #2193 ), #9137, .F. ) ;
#3516=CARTESIAN_POINT ( 'NONE',  ( -0.5291093370860696643, 13.28508303421404158, 38.99834356000749125 ) ) ;
#3519=B_SPLINE_CURVE_WITH_KNOTS ( 'NONE', 3,
 ( #9510, #1945, #4968, #5805 ),
 .UNSPECIFIED., .F., .F.,
 ( 4, 4 ),
 ( 0.000000000000000000, 0.003679109433542032855 ),
 .UNSPECIFIED. ) ;
#3528=CARTESIAN_POINT ( 'NONE',  ( 6.000000000000007994, -15.00000000000000000, 26.32489316217636954 ) ) ;
#3545=CARTESIAN_POINT ( 'NONE',  ( -11.07761026121387538, -4.999999999999996447, 37.39366993089406321 ) ) ;
#3552=CIRCLE ( 'NONE', #7342, 28.99999999999995026 ) ;
#3553=ORIENTED_EDGE ( 'NONE', *, *, #3907, .T. ) ;
#3555=CARTESIAN_POINT ( 'NONE',  ( 0.2508212505825567207, -9.470617022380011463, 39.52758568340708933 ) ) ;
#3563=CARTESIAN_POINT ( 'NONE',  ( 10.82166066357773637, 12.02267635125024015, 37.46937041031875992 ) ) ;
#3571=CLOSED_SHELL ( 'NONE', ( #3591, #5739, #3975, #8531, #4457, #4293, #4762, #5177, #4016, #4192, #6841, #7211, #7353, #9723, #541, #8488, #4217, #118, #3098, #2314, #2016, #5809, #4440, #9679, #2383, #6604, #1171, #292, #4441, #3756, #3515, #5482, #6061, #705, #4939, #7999, #9271, #386 ) ) ;
#3573=CARTESIAN_POINT ( 'NONE',  ( -3.849165636106636423, 12.55126050286880357, 38.86455347263002835 ) ) ;
#3591=ADVANCED_FACE ( 'NONE', ( #253 ), #2711, .T. ) ;
#3592=EDGE_LOOP ( 'NONE', ( #6104, #9357, #6808, #4126 ) ) ;
#3594=DIRECTION ( 'NONE',  ( 0.000000000000000000, 0.000000000000000000, -1.000000000000000000 ) ) ;
#3597=EDGE_CURVE ( 'NONE', #2973, #1345, #8242, .T. ) ;
#3602=CARTESIAN_POINT ( 'NONE',  ( -11.07761026121418269, -14.99999999999999645, 37.39366993089506508 ) ) ;
#3607=CARTESIAN_POINT ( 'NONE',  ( 8.665545440270191691, 8.296323355523078646, 42.03691472828050024 ) ) ;
#3612=CARTESIAN_POINT ( 'NONE',  ( 6.000000000000001776, 30.00000000000000000, -26.32489316217636954 ) ) ;
#3616=CARTESIAN_POINT ( 'NONE',  ( -1.355205547380036402, 13.21018532110894128, 38.98542963915694770 ) ) ;
#3618=FACE_OUTER_BOUND ( 'NONE', #8900, .T. ) ;
#3621=ORIENTED_EDGE ( 'NONE', *, *, #6046, .T. ) ;
#3630=EDGE_CURVE ( 'NONE', #5938, #9184, #992, .T. ) ;
#3637=DIRECTION ( 'NONE',  ( 0.000000000000000000, -1.000000000000000000, 0.000000000000000000 ) ) ;
#3638=CARTESIAN_POINT ( 'NONE',  ( 6.000000000000007994, -15.00000000000000000, 26.32489316217636954 ) ) ;
#3646=CARTESIAN_POINT ( 'NONE',  ( 4.817195445441472934, -15.00000000000000000, 29.05788463129285049 ) ) ;
#3647=ORIENTED_EDGE ( 'NONE', *, *, #5473, .T. ) ;
#3654=CARTESIAN_POINT ( 'NONE',  ( -8.237197373723139648, -4.999999999999998224, 27.80554943579302574 ) ) ;
#3655=FACE_OUTER_BOUND ( 'NONE', #7117, .T. ) ;
#3657=CARTESIAN_POINT ( 'NONE',  ( 9.365275055118548408, 6.895755298401112121, 38.01574831787047515 ) ) ;
#3666=VERTEX_POINT ( 'NONE', #8442 ) ;
#3667=CARTESIAN_POINT ( 'NONE',  ( -1.077604443879617291, 13.24265641225903600, 38.99104434882794834 ) ) ;
#3668=FACE_OUTER_BOUND ( 'NONE', #1425, .T. ) ;
#3675=FACE_OUTER_BOUND ( 'NONE', #1116, .T. ) ;
#3687=CARTESIAN_POINT ( 'NONE',  ( 5.488653208922126048, -15.00000000000000000, 28.77476281181572304 ) ) ;
#3689=EDGE_CURVE ( 'NONE', #7606, #2973, #4740, .T. ) ;
#3697=CARTESIAN_POINT ( 'NONE',  ( 10.07569075260316716, -15.00000000000064304, 37.15884857061433166 ) ) ;
#3698=ORIENTED_EDGE ( 'NONE', *, *, #3455, .F. ) ;
#3705=CARTESIAN_POINT ( 'NONE',  ( 8.477986360292581125, -2.018403734026263496, 42.12315275765950418 ) ) ;
#3713=ORIENTED_EDGE ( 'NONE', *, *, #6046, .F. ) ;
#3721=CARTESIAN_POINT ( 'NONE',  ( 0.000000000000000000, -4.999999999999997335, 0.000000000000000000 ) ) ;
#3736=EDGE_CURVE ( 'NONE', #6350, #1456, #2841, .T. ) ;
#3739=CARTESIAN_POINT ( 'NONE',  ( 0.000000000000000000, 13.29485247664129766, 300.0000000000000000 ) ) ;
#3749=DIRECTION ( 'NONE',  ( 0.000000000000000000, -0.000000000000000000, -1.000000000000000000 ) ) ;
#3750=CARTESIAN_POINT ( 'NONE',  ( 9.221621761046556287, -6.210574730312896641, 37.98076581590148493 ) ) ;
#3751=VERTEX_POINT ( 'NONE', #5128 ) ;
#3753=CARTESIAN_POINT ( 'NONE',  ( 0.02451486836956002016, 18.29482697815588566, 38.99999229514322252 ) ) ;
#3755=CARTESIAN_POINT ( 'NONE',  ( 12.11803679389154453, 9.485944279750869512, 37.06999036926945479 ) ) ;
#3756=ADVANCED_FACE ( 'NONE', ( #7197 ), #629, .F. ) ;
#3771=UNCERTAINTY_MEASURE_WITH_UNIT (LENGTH_MEASURE( 1.000000000000000082E-05 ), #4528, 'distance_accuracy_value', 'NONE');
#3776=CARTESIAN_POINT ( 'NONE',  ( 1.221566888952841201E-22, 27.99999999999992184, -31.00000000000000711 ) ) ;
#3788=DIRECTION ( 'NONE',  ( -0.000000000000000000, -0.000000000000000000, 1.000000000000000000 ) ) ;
#3800=CARTESIAN_POINT ( 'NONE',  ( 6.498172386907730136, -14.99999999999968381, 36.82545492661441955 ) ) ;
#3804=CARTESIAN_POINT ( 'NONE',  ( -6.000000000000005329, 28.28385863652523824, -30.12488991936162108 ) ) ;
#3806=CARTESIAN_POINT ( 'NONE',  ( 9.998641156849346956, 2.615690621352292133, 41.36497489834112429 ) ) ;
#3811=CARTESIAN_POINT ( 'NONE',  ( 0.000000000000000000, -4.999999999999999112, -29.00000000000001776 ) ) ;
#3817=B_SPLINE_CURVE_WITH_KNOTS ( 'NONE', 3,
 ( #9057, #3210, #954, #3967, #7676, #4761, #2325, #6958, #9114, #808, #3818, #6083, #6221, #6129, #8509, #6915, #3922, #9254, #2467, #5503, #6761, #1547, #1739, #20 ),
 .UNSPECIFIED., .F., .F.,
 ( 4, 2, 2, 2, 2, 2, 2, 2, 2, 2, 2, 4 ),
 ( 0.04762592066223522019, 0.04960947359156670650, 0.05060125005623244271, 0.05159302652089818586, 0.05357657945022965829, 0.05556013237956113071, 0.05655190884422686692, 0.05754368530889261008, 0.05952723823822408250, 0.06051901470288982565, 0.06151079116755556186, 0.06349434409688703429 ),
 .UNSPECIFIED. ) ;
#3818=CARTESIAN_POINT ( 'NONE',  ( -7.536685575068442056, -3.308866890532546012, 42.52863964422461862 ) ) ;
#3821=CARTESIAN_POINT ( 'NONE',  ( -2.587326571347316140, -9.215009914112087586, 39.41319473361446057 ) ) ;
#3825=CARTESIAN_POINT ( 'NONE',  ( -4.324486265735497881, -10.89814862554769803, 38.76179163200221467 ) ) ;
#3833=EDGE_CURVE ( 'NONE', #1089, #4910, #4450, .T. ) ;
#3836=CARTESIAN_POINT ( 'NONE',  ( 9.460130474090460595, 0.03677082304110015909, 41.64927532210272432 ) ) ;
#3840=CARTESIAN_POINT ( 'NONE',  ( -4.822163095725295889, -14.99999999999999822, 29.05566526170479591 ) ) ;
#3847=CARTESIAN_POINT ( 'NONE',  ( -31.00000000000000711, -15.00000000000000000, -5.999999999999996447 ) ) ;
#3850=LINE ( 'NONE', #7651, #1464 ) ;
#3851=CARTESIAN_POINT ( 'NONE',  ( 1.250417070894209948, -15.00000000000000000, 30.42002409700546650 ) ) ;
#3857=CARTESIAN_POINT ( 'NONE',  ( 9.680593967938868616, 5.886190330938374515, 41.53534638657208689 ) ) ;
#3867=CARTESIAN_POINT ( 'NONE',  ( -10.00000000000001599, 3.294852476658805873, 41.36423575989289247 ) ) ;
#3891=CARTESIAN_POINT ( 'NONE',  ( 3.551870781420234824, -6.058861246625666830, 43.67865056495266884 ) ) ;
#3894=FACE_OUTER_BOUND ( 'NONE', #8720, .T. ) ;
#3907=EDGE_CURVE ( 'NONE', #2298, #577, #2341, .T. ) ;
#3910=FACE_OUTER_BOUND ( 'NONE', #1208, .T. ) ;
#3913=CARTESIAN_POINT ( 'NONE',  ( 5.006257199294086746, -5.386139767686431767, 43.36232512974734021 ) ) ;
#3917=PLANE ( 'NONE',  #5759 ) ;
#3922=CARTESIAN_POINT ( 'NONE',  ( -4.486453089411146067, -5.666157368122981097, 43.49188059297183173 ) ) ;
#3925=CARTESIAN_POINT ( 'NONE',  ( -4.080223084771134268, -8.820719837204659797, 39.23376499704423281 ) ) ;
#3928=CARTESIAN_POINT ( 'NONE',  ( -1.339611196910782231, -6.636669372976692571, 43.96470529402514416 ) ) ;
#3938=CARTESIAN_POINT ( 'NONE',  ( 3.229357168250672760, 17.86321051590875442, 38.87085120031289875 ) ) ;
#3946=EDGE_CURVE ( 'NONE', #6269, #8266, #1617, .T. ) ;
#3948=DIRECTION ( 'NONE',  ( -0.000000000000000000, -1.000000000000000000, -0.000000000000000000 ) ) ;
#3955=CARTESIAN_POINT ( 'NONE',  ( -0.01963426291157483600, -6.705128248126140278, 43.99999014335539016 ) ) ;
#3967=CARTESIAN_POINT ( 'NONE',  ( -9.738952295719967012, 1.000838298946814087, 41.50427199400585465 ) ) ;
#3975=ADVANCED_FACE ( 'NONE', ( #3894 ), #1446, .T. ) ;
#3977=CARTESIAN_POINT ( 'NONE',  ( -7.783452355770943853, -8.875924410859513003, 38.21717263769323836 ) ) ;
#3978=DIRECTION ( 'NONE',  ( 0.000000000000000000, 0.000000000000000000, -1.000000000000000000 ) ) ;
#3979=AXIS2_PLACEMENT_3D ( 'NONE', #7947, #8737, #1373 ) ;
#3988=DIRECTION ( 'NONE',  ( 0.000000000000000000, 0.000000000000000000, 1.000000000000000000 ) ) ;
#3994=CARTESIAN_POINT ( 'NONE',  ( -18.51991245392837371, 3.294852476641298988, 294.6136752714472777 ) ) ;
#3995=ORIENTED_EDGE ( 'NONE', *, *, #9217, .F. ) ;
#4010=EDGE_CURVE ( 'NONE', #9635, #2374, #3403, .T. ) ;
#4012=CARTESIAN_POINT ( 'NONE',  ( 28.37252191822216218, 30.00000000000000000, 6.000000000000000000 ) ) ;
#4016=ADVANCED_FACE ( 'NONE', ( #4040 ), #6932, .F. ) ;
#4017=VECTOR ( 'NONE', #5130, 1000.000000000000000 ) ;
#4026=CARTESIAN_POINT ( 'NONE',  ( -10.56205462419233498, -5.828843216915552183, 37.54361741745486114 ) ) ;
#4035=CIRCLE ( 'NONE', #719, 10.00000000000000178 ) ;
#4040=FACE_OUTER_BOUND ( 'NONE', #3592, .T. ) ;
#4047=DIRECTION ( 'NONE',  ( -0.000000000000000000, 1.000000000000000000, -0.000000000000000000 ) ) ;
#4052=VERTEX_POINT ( 'NONE', #1020 ) ;
#4053=CARTESIAN_POINT ( 'NONE',  ( -6.000000000000005329, 27.42469319230600533, -31.00000000000000711 ) ) ;
#4058=CARTESIAN_POINT ( 'NONE',  ( 3.525292369978886065, -6.068895536008623637, 43.68349390364525675 ) ) ;
#4069=CARTESIAN_POINT ( 'NONE',  ( -5.999999999999998224, 30.00000000000000000, 31.00000000000000711 ) ) ;
#4072=ORIENTED_EDGE ( 'NONE', *, *, #4085, .F. ) ;
#4074=VERTEX_POINT ( 'NONE', #925 ) ;
#4076=CARTESIAN_POINT ( 'NONE',  ( -11.54630107002959427, -4.206870269394932471, 37.25503203836519361 ) ) ;
#4082=ORIENTED_EDGE ( 'NONE', *, *, #2276, .T. ) ;
#4085=EDGE_CURVE ( 'NONE', #5016, #3264, #5614, .T. ) ;
#4098=CARTESIAN_POINT ( 'NONE',  ( 6.000000000000001776, -15.00000000000000000, -26.32489316217636954 ) ) ;
#4099=CARTESIAN_POINT ( 'NONE',  ( 6.000000000000007994, 30.00000000000000000, 26.32489316217636954 ) ) ;
#4101=CARTESIAN_POINT ( 'NONE',  ( -13.22790787108309907, 4.939837902798808855, 36.68820129006189745 ) ) ;
#4104=AXIS2_PLACEMENT_3D ( 'NONE', #6141, #3081, #2337 ) ;
#4105=CIRCLE ( 'NONE', #7894, 13.53485947486097984 ) ;
#4107=CARTESIAN_POINT ( 'NONE',  ( 5.496802345886652397, -5.097331429848454221, 38.70186493977237063 ) ) ;
#4112=CARTESIAN_POINT ( 'NONE',  ( 6.000000000000007994, -10.00000000000000533, 26.32489316217636954 ) ) ;
#4126=ORIENTED_EDGE ( 'NONE', *, *, #8055, .T. ) ;
#4127=CARTESIAN_POINT ( 'NONE',  ( -13.11784307232190372, 5.787500145060168855, 36.72779070367025156 ) ) ;
#4129=AXIS2_PLACEMENT_3D ( 'NONE', #3528, #2785, #1856 ) ;
#4144=EDGE_LOOP ( 'NONE', ( #7901, #4905, #7166, #3259 ) ) ;
#4150=CARTESIAN_POINT ( 'NONE',  ( -11.73250938807055377, -3.886762146447892086, 37.19966069614565640 ) ) ;
#4161=ORIENTED_EDGE ( 'NONE', *, *, #1418, .T. ) ;
#4162=DIRECTION ( 'NONE',  ( 0.2840412887490734728, 0.000000000000000000, 0.9588120495101037921 ) ) ;
#4163=ORIENTED_EDGE ( 'NONE', *, *, #1180, .T. ) ;
#4175=CARTESIAN_POINT ( 'NONE',  ( -9.664726846066640675, 0.7061636768653499763, 41.54343935902185336 ) ) ;
#4189=DIRECTION ( 'NONE',  ( -0.000000000000000000, 1.000000000000000000, -0.000000000000000000 ) ) ;
#4192=ADVANCED_FACE ( 'NONE', ( #8125 ), #2636, .F. ) ;
#4201=CARTESIAN_POINT ( 'NONE',  ( -8.258691924487683522, 15.13224157323768182, 38.13012333692111611 ) ) ;
#4202=AXIS2_PLACEMENT_3D ( 'NONE', #6733, #2884, #6682 ) ;
#4206=AXIS2_PLACEMENT_3D ( 'NONE', #7617, #2265, #1542 ) ;
#4208=CARTESIAN_POINT ( 'NONE',  ( 0.000000000000000000, -15.00000000000000000, 0.000000000000000000 ) ) ;
#4211=CARTESIAN_POINT ( 'NONE',  ( -1.783504999752484332, -15.00000000000000000, 30.27207878768652805 ) ) ;
#4214=VECTOR ( 'NONE', #4895, 1000.000000000000000 ) ;
#4215=EDGE_CURVE ( 'NONE', #8266, #1456, #6291, .T. ) ;
#4216=( BOUNDED_SURFACE ( )  B_SPLINE_SURFACE ( 3, 2, ( 
 ( #2060, #3602, #2013 ),
 ( #6602, #6414, #9624 ),
 ( #2850, #2705, #4401 ),
 ( #5141, #4995, #5036 ),
 ( #458, #9441, #8150 ),
 ( #4301, #1921, #1971 ),
 ( #5086, #6511, #5783 ),
 ( #7957, #2803, #5682 ),
 ( #3454, #8047, #8097 ),
 ( #5728, #8700, #7253 ),
 ( #2104, #409, #1192 ),
 ( #4211, #4253, #7208 ),
 ( #6456, #9483, #5865 ),
 ( #8888, #7305, #503 ),
 ( #1331, #1287, #6563 ),
 ( #8005, #1240, #3500 ),
 ( #9586, #5822, #9531 ),
 ( #2758, #556, #3555 ),
 ( #4357, #2154, #9673 ),
 ( #2895, #843, #3044 ),
 ( #2246, #5385, #2951 ),
 ( #1427, #4448, #5185 ),
 ( #6744, #9138, #7559 ),
 ( #3851, #113, #5279 ),
 ( #4599, #789, #5 ),
 ( #6848, #693, #54 ),
 ( #8297, #741, #6004 ),
 ( #7605, #3096, #5335 ),
 ( #4547, #6110, #2306 ),
 ( #1526, #3800, #6798 ),
 ( #8343, #6056, #9091 ),
 ( #1580, #7453, #6647 ),
 ( #3646, #2353, #8942 ),
 ( #8394, #1626, #3750 ),
 ( #2996, #8193, #7408 ),
 ( #642, #3697, #9038 ),
 ( #6699, #5959, #5915 ),
 ( #4495, #9728, #8985 ) ),
 .UNSPECIFIED., .F., .F., .F. ) 
 B_SPLINE_SURFACE_WITH_KNOTS ( ( 4, 2, 2, 2, 2, 2, 2, 2, 2, 2, 2, 2, 2, 2, 2, 2, 2, 2, 4 ),
 ( 3, 3 ),
 ( 1.795438797635995343E-16, 0.002181780987149469723, 0.003272671480724114595, 0.004363561974298759902, 0.005454452467873405208, 0.006545342961448049647, 0.007636233455022694086, 0.008181678701810017607, 0.008727123948597339392, 0.008999846571991000285, 0.009272569195384661178, 0.009818014442171984699, 0.01036345968895930822, 0.01090890493574663000, 0.01199979542932127358, 0.01309068592289591888, 0.01418157641647056419, 0.01527246691004520776, 0.01745424789719449837 ),
 ( 0.000000000000000000, 1.000000000000000000 ),
 .UNSPECIFIED. ) 
 GEOMETRIC_REPRESENTATION_ITEM ( )  RATIONAL_B_SPLINE_SURFACE ( (
 ( 1.000000000000000000, 0.7071067811865473507, 1.000000000000000000),
 ( 1.000000000000000000, 0.7161513553615299621, 1.000000000000000000),
 ( 1.000000000000000000, 0.7261151885358542168, 1.000000000000000000),
 ( 1.000000000000000000, 0.7427909353351239696, 1.000000000000000000),
 ( 1.000000000000000000, 0.7486383365456040773, 1.000000000000000000),
 ( 1.000000000000000000, 0.7609590083029650343, 1.000000000000000000),
 ( 1.000000000000000000, 0.7674338186474088941, 1.000000000000000000),
 ( 1.000000000000000000, 0.7810218732661525776, 1.000000000000000000),
 ( 1.000000000000000000, 0.7881405391415673423, 1.000000000000000000),
 ( 1.000000000000000000, 0.8029038133575651104, 1.000000000000000000),
 ( 1.000000000000000000, 0.8105722495354327206, 1.000000000000000000),
 ( 1.000000000000000000, 0.8258428283520197200, 1.000000000000000000),
 ( 1.000000000000000000, 0.8335350131668984863, 1.000000000000000000),
 ( 1.000000000000000000, 0.8428590422713853059, 1.000000000000000000),
 ( 1.000000000000000000, 0.8455698979328197806, 1.000000000000000000),
 ( 1.000000000000000000, 0.8494339551369524122, 1.000000000000000000),
 ( 1.000000000000000000, 0.8505582715026442919, 1.000000000000000000),
 ( 1.000000000000000000, 0.8506061670060169888, 1.000000000000000000),
 ( 1.000000000000000000, 0.8503513266545774663, 1.000000000000000000),
 ( 1.000000000000000000, 0.8493382604359895893, 1.000000000000000000),
 ( 1.000000000000000000, 0.8485833736532394367, 1.000000000000000000),
 ( 1.000000000000000000, 0.8457164237044830779, 1.000000000000000000),
 ( 1.000000000000000000, 0.8430121088779416461, 1.000000000000000000),
 ( 1.000000000000000000, 0.8368088722261513013, 1.000000000000000000),
 ( 1.000000000000000000, 0.8333129582802408786, 1.000000000000000000),
 ( 1.000000000000000000, 0.8260259447890396789, 1.000000000000000000),
 ( 1.000000000000000000, 0.8222304458373403957, 1.000000000000000000),
 ( 1.000000000000000000, 0.8107652166501773117, 1.000000000000000000),
 ( 1.000000000000000000, 0.8030801492908825612, 1.000000000000000000),
 ( 1.000000000000000000, 0.7882884757859640601, 1.000000000000000000),
 ( 1.000000000000000000, 0.7811556660049406853, 1.000000000000000000),
 ( 1.000000000000000000, 0.7675411181467285404, 1.000000000000000000),
 ( 1.000000000000000000, 0.7610538784716394112, 1.000000000000000000),
 ( 1.000000000000000000, 0.7487101099141471039, 1.000000000000000000),
 ( 1.000000000000000000, 0.7428520250537596903, 1.000000000000000000),
 ( 1.000000000000000000, 0.7261465437174193793, 1.000000000000000000),
 ( 1.000000000000000000, 0.7161659583961312858, 1.000000000000000000),
 ( 1.000000000000000000, 0.7071067811865477948, 1.000000000000000000) ) ) 
 REPRESENTATION_ITEM ( '' )  SURFACE ( )  );
#4217=ADVANCED_FACE ( 'NONE', ( #483 ), #6393, .F. ) ;
#4223=ORIENTED_EDGE ( 'NONE', *, *, #6311, .F. ) ;
#4226=AXIS2_PLACEMENT_3D ( 'NONE', #8824, #2047, #1273 ) ;
#4228=CARTESIAN_POINT ( 'NONE',  ( -7.530772855371751895, -3.328027317286678777, 38.39592399675708378 ) ) ;
#4237=CARTESIAN_POINT ( 'NONE',  ( 12.77996869406904068, 7.481990194735835153, 36.84712280227347492 ) ) ;
#4239=LINE ( 'NONE', #486, #6223 ) ;
#4243=CARTESIAN_POINT ( 'NONE',  ( 9.916385959428817287, 4.627893224472521716, 41.40953687719313336 ) ) ;
#4248=CARTESIAN_POINT ( 'NONE',  ( 3.538670939391739712, -8.984539127871803643, 39.30863205750186751 ) ) ;
#4249=EDGE_CURVE ( 'NONE', #4378, #9481, #3519, .T. ) ;
#4253=CARTESIAN_POINT ( 'NONE',  ( -3.866809454646866318, -15.00000000000031442, 36.77917012741243497 ) ) ;
#4259=CARTESIAN_POINT ( 'NONE',  ( 8.371299763093835722, 8.807943335447152577, 38.23376413749986114 ) ) ;
#4265=EDGE_CURVE ( 'NONE', #4910, #1089, #4105, .T. ) ;
#4268=ORIENTED_EDGE ( 'NONE', *, *, #7755, .F. ) ;
#4271=CARTESIAN_POINT ( 'NONE',  ( -3.570894301289286421, 12.65974171353586719, 38.88496779480359322 ) ) ;
#4273=CARTESIAN_POINT ( 'NONE',  ( -5.999999999999998224, 28.28385863652524179, 30.12488991936162464 ) ) ;
#4276=ORIENTED_EDGE ( 'NONE', *, *, #3630, .F. ) ;
#4283=FACE_OUTER_BOUND ( 'NONE', #9401, .T. ) ;
#4293=ADVANCED_FACE ( 'NONE', ( #8771 ), #2039, .T. ) ;
#4301=CARTESIAN_POINT ( 'NONE',  ( -4.822208557843039145, -15.00000000000000000, 29.05578429771093951 ) ) ;
#4307=CARTESIAN_POINT ( 'NONE',  ( 2.211399979663802196, 18.09417943208245205, 38.93963529505569454 ) ) ;
#4316=CARTESIAN_POINT ( 'NONE',  ( -5.282492592870707604, 11.79197944368125839, 43.28262095644331708 ) ) ;
#4318=PLANE ( 'NONE',  #4827 ) ;
#4329=FACE_OUTER_BOUND ( 'NONE', #2123, .T. ) ;
#4336=B_SPLINE_CURVE_WITH_KNOTS ( 'NONE', 3,
 ( #7044, #4516, #1821, #2268, #6815, #2322, #8587, #2211, #9743, #301, #2966, #1034, #9003, #131, #3296, #4616, #7473, #7572, #8358, #1545, #6305, #859, #2544, #72, #8315, #3867 ),
 .UNSPECIFIED., .F., .F.,
 ( 4, 2, 2, 2, 2, 2, 2, 2, 2, 2, 2, 2, 4 ),
 ( 0.03173335151219601469, 0.03272663708407346633, 0.03371992265595091104, 0.03570649379970581433, 0.03669977937158326597, 0.03769306494346071068, 0.03967963608721561397, 0.04067292165909306562, 0.04166620723097052420, 0.04365277837472542055, 0.04563934951848032384, 0.04663263509035776855, 0.04762592066223522019 ),
 .UNSPECIFIED. ) ;
#4338=TOROIDAL_SURFACE ( 'NONE', #8272, 29.00000000000001776, 10.00000000000000000 ) ;
#4342=CARTESIAN_POINT ( 'NONE',  ( 2.649740526188390621, 12.96017046470857359, 43.83099598276683651 ) ) ;
#4357=CARTESIAN_POINT ( 'NONE',  ( 0.1750943534869517371, -15.00000000000000178, 30.57953220782976800 ) ) ;
#4362=CARTESIAN_POINT ( 'NONE',  ( 0.000000000000000000, 30.00000000000000000, 0.000000000000000000 ) ) ;
#4364=CARTESIAN_POINT ( 'NONE',  ( 0.6754392200130907575, 13.27748550001718897, 43.99110106382870811 ) ) ;
#4373=CARTESIAN_POINT ( 'NONE',  ( -4.125509516341439031, 12.41002393623410605, 43.56504187369129255 ) ) ;
#4374=DIRECTION ( 'NONE',  ( -1.000000000000000000, 0.000000000000000000, 0.000000000000000000 ) ) ;
#4378=VERTEX_POINT ( 'NONE', #767 ) ;
#4379=CARTESIAN_POINT ( 'NONE',  ( 26.32489316217636954, 30.00000000000000000, -6.000000000000006217 ) ) ;
#4383=( NAMED_UNIT ( * ) PLANE_ANGLE_UNIT ( ) SI_UNIT ( $, .RADIAN. ) );
#4393=EDGE_CURVE ( 'NONE', #5506, #7120, #7299, .T. ) ;
#4396=PLANE ( 'NONE',  #8116 ) ;
#4401=CARTESIAN_POINT ( 'NONE',  ( -10.24028423210522476, -5.542393513087790602, 37.65233335542363591 ) ) ;
#4406=CARTESIAN_POINT ( 'NONE',  ( 11.52123655141487113, 10.79705879502866139, 37.25999260019175097 ) ) ;
#4413=CARTESIAN_POINT ( 'NONE',  ( -1.720948704681326991, 18.17687923655758553, 38.96445573820884078 ) ) ;
#4437=CARTESIAN_POINT ( 'NONE',  ( -31.00000000000000711, 27.80235549540589801, -4.012532818320189598 ) ) ;
#4440=ADVANCED_FACE ( 'NONE', ( #6770 ), #27, .T. ) ;
#4441=ADVANCED_FACE ( 'NONE', ( #3675 ), #2933, .T. ) ;
#4447=CARTESIAN_POINT ( 'NONE',  ( 0.000000000000000000, -10.00000000000000533, 0.000000000000000000 ) ) ;
#4448=CARTESIAN_POINT ( 'NONE',  ( 1.689983091256852976, -15.00000000000062883, 36.76756119980281312 ) ) ;
#4450=CIRCLE ( 'NONE', #3979, 13.53485947486097984 ) ;
#4457=ADVANCED_FACE ( 'NONE', ( #7214 ), #3244, .F. ) ;
#4466=CARTESIAN_POINT ( 'NONE',  ( -2.185593797502169089, 13.07767852523060803, 38.96206052328675185 ) ) ;
#4480=ORIENTED_EDGE ( 'NONE', *, *, #2130, .T. ) ;
#4483=CARTESIAN_POINT ( 'NONE',  ( 8.237197373723128990, -15.00000000000000000, 27.80554943579302574 ) ) ;
#4490=CARTESIAN_POINT ( 'NONE',  ( 31.00000000000000711, 27.42469319230600533, -6.000000000000006217 ) ) ;
#4495=CARTESIAN_POINT ( 'NONE',  ( 8.237197373723113003, -15.00000000000000000, 27.80554943579302929 ) ) ;
#4497=ORIENTED_EDGE ( 'NONE', *, *, #8395, .T. ) ;
#4502=CARTESIAN_POINT ( 'NONE',  ( 9.461646124974400607, 0.04132284101285077504, 41.64849753988102066 ) ) ;
#4504=PRODUCT_CONTEXT ( 'NONE', #8652, 'mechanical' ) ;
#4508=EDGE_CURVE ( 'NONE', #3264, #9481, #2460, .T. ) ;
#4509=CARTESIAN_POINT ( 'NONE',  ( -5.999999999999998224, -10.00000000000000533, 31.00000000000000711 ) ) ;
#4516=CARTESIAN_POINT ( 'NONE',  ( -0.3130905416343935377, 13.29544676968441053, 44.00030389938851272 ) ) ;
#4528=( LENGTH_UNIT ( ) NAMED_UNIT ( * ) SI_UNIT ( .MILLI., .METRE. ) );
#4547=CARTESIAN_POINT ( 'NONE',  ( 2.800868546665862269, -15.00000000000000000, 29.90216386052837549 ) ) ;
#4549=DIRECTION ( 'NONE',  ( -0.000000000000000000, 1.000000000000000000, -0.000000000000000000 ) ) ;
#4552=CARTESIAN_POINT ( 'NONE',  ( 9.839714455520448766, 5.126572604364064034, 37.89933748290150817 ) ) ;
#4556=DIRECTION ( 'NONE',  ( -1.000000000000000000, -0.000000000000000000, -0.000000000000000000 ) ) ;
#4559=ORIENTED_EDGE ( 'NONE', *, *, #4393, .T. ) ;
#4560=CARTESIAN_POINT ( 'NONE',  ( -0.9994180975881532536, 27.99999999999992895, -31.00000000000001066 ) ) ;
#4562=DIRECTION ( 'NONE',  ( 0.000000000000000000, -1.000000000000000000, 0.000000000000000000 ) ) ;
#4568=CARTESIAN_POINT ( 'NONE',  ( -0.02206928620401079830, -9.470079073673241865, 39.52734620791224529 ) ) ;
#4573=CARTESIAN_POINT ( 'NONE',  ( -1.936180212574767801, -6.526933022534523232, 38.96892306166470377 ) ) ;
#4574=CARTESIAN_POINT ( 'NONE',  ( 0.000000000000000000, -10.00000000000000533, 0.000000000000000000 ) ) ;
#4588=CARTESIAN_POINT ( 'NONE',  ( -3.482141448764432212, -15.00000000000000000, 29.62376806748125446 ) ) ;
#4590=CARTESIAN_POINT ( 'NONE',  ( -5.999999999999998224, 30.00000000000000000, 28.37252191822216218 ) ) ;
#4593=CIRCLE ( 'NONE', #415, 27.00000000000000355 ) ;
#4599=CARTESIAN_POINT ( 'NONE',  ( 1.425420758115970354, -14.99999999999999822, 30.37403179307458601 ) ) ;
#4607=CARTESIAN_POINT ( 'NONE',  ( 13.20615709665468529, 1.297055670843870301, 36.69647536524409048 ) ) ;
#4609=VERTEX_POINT ( 'NONE', #2091 ) ;
#4610=LINE ( 'NONE', #2260, #6554 ) ;
#4615=ORIENTED_EDGE ( 'NONE', *, *, #7286, .T. ) ;
#4616=CARTESIAN_POINT ( 'NONE',  ( -7.921576059427342997, 9.406609150246151074, 42.36640274441228371 ) ) ;
#4622=CARTESIAN_POINT ( 'NONE',  ( 4.776122516674679455E-15, 19.99999999999982236, -39.00000000000002132 ) ) ;
#4637=CARTESIAN_POINT ( 'NONE',  ( 4.460510837761463065, -5.679267476043179386, 43.49797445894572689 ) ) ;
#4640=CARTESIAN_POINT ( 'NONE',  ( 2.805732460449232857, -15.00000000000000000, 29.91534241968305352 ) ) ;
#4645=CARTESIAN_POINT ( 'NONE',  ( -31.00000000000001066, 27.75862132583096553, 4.003261267919811850 ) ) ;
#4647=ORIENTED_EDGE ( 'NONE', *, *, #1288, .T. ) ;
#4655=CARTESIAN_POINT ( 'NONE',  ( 6.080049472934138777, -4.651243486359556201, 43.04620881594706105 ) ) ;
#4676=CARTESIAN_POINT ( 'NONE',  ( -3.485699947575983781, -11.18892459271980577, 38.84620403412360190 ) ) ;
#4688=CARTESIAN_POINT ( 'NONE',  ( 1.313076780747179484, 18.23965141680392321, 38.98324215956266414 ) ) ;
#4701=ORIENTED_EDGE ( 'NONE', *, *, #7565, .T. ) ;
#4704=CARTESIAN_POINT ( 'NONE',  ( 1.300547793265065533, -6.641803996390986953, 43.96733177750241595 ) ) ;
#4713=CARTESIAN_POINT ( 'NONE',  ( -2.083000153361134643, -9.308704936926149642, 39.45524585924379579 ) ) ;
#4714=ORIENTED_EDGE ( 'NONE', *, *, #4249, .T. ) ;
#4738=PRODUCT_DEFINITION_SHAPE ( 'NONE', 'NONE',  #8147 ) ;
#4740=LINE ( 'NONE', #4098, #3029 ) ;
#4761=CARTESIAN_POINT ( 'NONE',  ( -9.463197482281705319, 0.04576215439031022097, 41.64770477980678010 ) ) ;
#4762=ADVANCED_FACE ( 'NONE', ( #4283 ), #7281, .T. ) ;
#4763=ORIENTED_EDGE ( 'NONE', *, *, #8070, .T. ) ;
#4769=CARTESIAN_POINT ( 'NONE',  ( -9.999521393725496310, 3.638235021868027719, 41.36449609663748106 ) ) ;
#4772=AXIS2_PLACEMENT_3D ( 'NONE', #7595, #8384, #8334 ) ;
#4784=CARTESIAN_POINT ( 'NONE',  ( -31.00000000000000711, 27.42469319230600533, 6.000000000000009770 ) ) ;
#4787=FACE_OUTER_BOUND ( 'NONE', #7466, .T. ) ;
#4789=DIRECTION ( 'NONE',  ( 0.000000000000000000, 0.000000000000000000, -1.000000000000000000 ) ) ;
#4790=LINE ( 'NONE', #4099, #587 ) ;
#4794=EDGE_CURVE ( 'NONE', #9521, #7758, #5975, .T. ) ;
#4798=CARTESIAN_POINT ( 'NONE',  ( -0.02610464500743471528, -11.70511861050984947, 38.99999126342864741 ) ) ;
#4818=CARTESIAN_POINT ( 'NONE',  ( -9.745578801763752352, 1.029427285159154160, 41.50076718676587006 ) ) ;
#4822=EDGE_LOOP ( 'NONE', ( #2172, #266, #3229, #7371, #1484 ) ) ;
#4824=ORIENTED_EDGE ( 'NONE', *, *, #6477, .T. ) ;
#4825=DIRECTION ( 'NONE',  ( 0.000000000000000000, -1.000000000000000000, 0.000000000000000000 ) ) ;
#4827=AXIS2_PLACEMENT_3D ( 'NONE', #9693, #5202, #8210 ) ;
#4833=DIRECTION ( 'NONE',  ( -0.000000000000000000, 1.000000000000000000, -0.000000000000000000 ) ) ;
#4834=CIRCLE ( 'NONE', #569, 10.00000000000001599 ) ;
#4843=CARTESIAN_POINT ( 'NONE',  ( -13.30454745595961263, 3.637961880295645045, 36.66047841392798290 ) ) ;
#4844=DIRECTION ( 'NONE',  ( -0.000000000000000000, -1.000000000000000000, -0.000000000000000000 ) ) ;
#4846=DIRECTION ( 'NONE',  ( -1.000000000000000000, 0.000000000000000000, 0.000000000000000000 ) ) ;
#4853=CYLINDRICAL_SURFACE ( 'NONE', #6800, 10.00000000000001599 ) ;
#4861=CARTESIAN_POINT ( 'NONE',  ( -10.00092682600661398, 2.650786234224241422, 41.36373161509812491 ) ) ;
#4865=CARTESIAN_POINT ( 'NONE',  ( 31.00000000000000711, 30.00000000000000000, 6.000000000000000000 ) ) ;
#4872=CARTESIAN_POINT ( 'NONE',  ( 11.82328533550226446, -3.573622092248616600, 37.16487311033493768 ) ) ;
#4877=ORIENTED_EDGE ( 'NONE', *, *, #5797, .F. ) ;
#4878=CARTESIAN_POINT ( 'NONE',  ( 0.02765780018129053094, 18.29482697815594605, 43.99999130734107666 ) ) ;
#4895=DIRECTION ( 'NONE',  ( 1.000000000000000000, 0.000000000000000000, 0.000000000000000000 ) ) ;
#4905=ORIENTED_EDGE ( 'NONE', *, *, #5824, .T. ) ;
#4910=VERTEX_POINT ( 'NONE', #1114 ) ;
#4911=CARTESIAN_POINT ( 'NONE',  ( -6.620562216048003989, -4.206768621063721625, 42.86638935774112014 ) ) ;
#4913=VECTOR ( 'NONE', #9700, 1000.000000000000000 ) ;
#4916=ORIENTED_EDGE ( 'NONE', *, *, #197, .T. ) ;
#4917=CARTESIAN_POINT ( 'NONE',  ( -26.32489316217637665, -10.00000000000000533, -5.999999999999997335 ) ) ;
#4918=VERTEX_POINT ( 'NONE', #4917 ) ;
#4922=CARTESIAN_POINT ( 'NONE',  ( 11.68706106293763369, -3.864370397872626928, 37.20800715665480851 ) ) ;
#4930=ORIENTED_EDGE ( 'NONE', *, *, #3946, .T. ) ;
#4937=CARTESIAN_POINT ( 'NONE',  ( -12.40769890286448529, 8.723482751359334486, 36.97414555372668588 ) ) ;
#4939=ADVANCED_FACE ( 'NONE', ( #3434 ), #3140, .T. ) ;
#4950=CARTESIAN_POINT ( 'NONE',  ( 5.533140936547730426, 11.68019839214159639, 38.70043871012786241 ) ) ;
#4958=CARTESIAN_POINT ( 'NONE',  ( -9.727440649738706924, -6.942074567273613717, 37.76869895888170703 ) ) ;
#4960=DIRECTION ( 'NONE',  ( -0.000000000000000000, 1.000000000000000000, -0.000000000000000000 ) ) ;
#4962=AXIS2_PLACEMENT_3D ( 'NONE', #8582, #4047, #6986 ) ;
#4966=ORIENTED_EDGE ( 'NONE', *, *, #5797, .T. ) ;
#4968=CARTESIAN_POINT ( 'NONE',  ( -30.12488991936162464, 28.28385863652524179, -5.999999999999996447 ) ) ;
#4970=DIRECTION ( 'NONE',  ( -0.000000000000000000, 1.000000000000000000, -0.000000000000000000 ) ) ;
#4979=VECTOR ( 'NONE', #1147, 1000.000000000000000 ) ;
#4984=CARTESIAN_POINT ( 'NONE',  ( 0.000000000000000000, -10.00000000000000533, 0.000000000000000000 ) ) ;
#4986=EDGE_CURVE ( 'NONE', #915, #9635, #487, .T. ) ;
#4992=DIRECTION ( 'NONE',  ( 0.000000000000000000, 0.000000000000000000, 1.000000000000000000 ) ) ;
#4995=CARTESIAN_POINT ( 'NONE',  ( -9.151040477096435311, -15.00000000000093614, 37.02450192303366094 ) ) ;
#4998=EDGE_CURVE ( 'NONE', #8477, #5016, #3186, .T. ) ;
#5002=CARTESIAN_POINT ( 'NONE',  ( 7.533895508403737118, 9.914173740682880265, 38.39536267294633376 ) ) ;
#5008=VECTOR ( 'NONE', #8183, 1000.000000000000000 ) ;
#5010=CARTESIAN_POINT ( 'NONE',  ( -5.485052425114111507, 16.96760966600532683, 38.61446893340349362 ) ) ;
#5016=VERTEX_POINT ( 'NONE', #8485 ) ;
#5019=PLANE ( 'NONE',  #4129 ) ;
#5024=CARTESIAN_POINT ( 'NONE',  ( 0.3492264405225555812, 13.29422555222517843, 43.99967941412595707 ) ) ;
#5029=DIRECTION ( 'NONE',  ( 0.000000000000000000, 0.000000000000000000, -1.000000000000000000 ) ) ;
#5036=CARTESIAN_POINT ( 'NONE',  ( -9.491181639781968826, -6.034149515792501361, 37.89378918816769470 ) ) ;
#5057=CARTESIAN_POINT ( 'NONE',  ( -7.036077784066177010, 10.44445367756955534, 38.48139619194807182 ) ) ;
#5058=DIRECTION ( 'NONE',  ( 0.000000000000000000, 0.000000000000000000, -1.000000000000000000 ) ) ;
#5059=CARTESIAN_POINT ( 'NONE',  ( 0.000000000000000000, -4.999999999999999112, 0.000000000000000000 ) ) ;
#5061=EDGE_LOOP ( 'NONE', ( #7097, #4916, #9257, #4877 ) ) ;
#5067=CARTESIAN_POINT ( 'NONE',  ( 0.000000000000000000, 3.294852476641296768, 300.0000000000000000 ) ) ;
#5073=VERTEX_POINT ( 'NONE', #4590 ) ;
#5075=CARTESIAN_POINT ( 'NONE',  ( 9.866687305369380212, 4.955150770795770931, 41.43633485533133864 ) ) ;
#5078=CARTESIAN_POINT ( 'NONE',  ( -6.000000000000005329, 30.00000000000000000, -26.32489316217636954 ) ) ;
#5079=CARTESIAN_POINT ( 'NONE',  ( 0.000000000000000000, 30.00000000000000000, 0.000000000000000000 ) ) ;
#5086=CARTESIAN_POINT ( 'NONE',  ( -4.487157684392466095, -15.00000000000000000, 29.19769096421646282 ) ) ;
#5095=CARTESIAN_POINT ( 'NONE',  ( 6.062272466284918337, 11.31083119101153578, 38.63159523596766576 ) ) ;
#5105=CARTESIAN_POINT ( 'NONE',  ( -7.729170831334030822, 9.683805115199277225, 38.35949281304758074 ) ) ;
#5128=CARTESIAN_POINT ( 'NONE',  ( -5.999999999999998224, 30.00000000000000000, 26.32489316217636954 ) ) ;
#5130=DIRECTION ( 'NONE',  ( 1.000000000000000000, 0.000000000000000000, 0.000000000000000000 ) ) ;
#5132=CIRCLE ( 'NONE', #1657, 28.99999999999995026 ) ;
#5141=CARTESIAN_POINT ( 'NONE',  ( -5.832239843001731927, -15.00000000000000000, 28.64283837909960795 ) ) ;
#5148=CARTESIAN_POINT ( 'NONE',  ( 1.772214115361161912, 18.16925905107996186, 38.96216795829242585 ) ) ;
#5158=CARTESIAN_POINT ( 'NONE',  ( -1.624225145205289156, 13.16760741291165537, 43.93520348923563290 ) ) ;
#5168=DIRECTION ( 'NONE',  ( 1.000000000000000000, 0.000000000000000000, 0.000000000000000000 ) ) ;
#5175=LINE ( 'NONE', #9473, #5008 ) ;
#5177=ADVANCED_FACE ( 'NONE', ( #5708 ), #6395, .F. ) ;
#5185=CARTESIAN_POINT ( 'NONE',  ( 2.108145055611895469, -9.304652320644109409, 39.45342799411329793 ) ) ;
#5192=CARTESIAN_POINT ( 'NONE',  ( 10.54343430594074960, -5.895781167747204954, 37.55119601223130843 ) ) ;
#5200=ORIENTED_EDGE ( 'NONE', *, *, #7223, .T. ) ;
#5202=DIRECTION ( 'NONE',  ( -0.000000000000000000, 0.000000000000000000, 1.000000000000000000 ) ) ;
#5204=AXIS2_PLACEMENT_3D ( 'NONE', #7028, #6283, #9310 ) ;
#5213=SHAPE_REPRESENTATION ( 'Lever with a Die for Securing the Metal Body', ( #6314 ), #2196 ) ;
#5218=ORIENTED_EDGE ( 'NONE', *, *, #9565, .F. ) ;
#5219=CARTESIAN_POINT ( 'NONE',  ( -0.01963426291156584666, -6.705128248126137613, 43.99999014335539016 ) ) ;
#5224=CARTESIAN_POINT ( 'NONE',  ( -0.6447393712377219588, 18.29485247664131364, 39.00000000000001421 ) ) ;
#5229=CARTESIAN_POINT ( 'NONE',  ( -31.00000000000000711, 27.42469319230600533, 6.000000000000009770 ) ) ;
#5238=CARTESIAN_POINT ( 'NONE',  ( 8.737909304966237301, 8.199549718101609486, 38.15650413348530634 ) ) ;
#5247=ORIENTED_EDGE ( 'NONE', *, *, #3689, .F. ) ;
#5259=CARTESIAN_POINT ( 'NONE',  ( -6.000000000000005329, -15.00000000000000000, -31.00000000000000711 ) ) ;
#5264=ORIENTED_EDGE ( 'NONE', *, *, #5522, .F. ) ;
#5266=CARTESIAN_POINT ( 'NONE',  ( 10.00000000000001599, 3.294852476638864491, 41.36423575989288537 ) ) ;
#5268=CARTESIAN_POINT ( 'NONE',  ( -0.3732932347937627515, -15.00000000000000000, 30.58137713278830105 ) ) ;
#5279=CARTESIAN_POINT ( 'NONE',  ( 3.456999781945461425, -9.004789367952092505, 39.31782667389276043 ) ) ;
#5289=CARTESIAN_POINT ( 'NONE',  ( 9.900265737266146004, 4.761116128428549921, 37.88407853222265231 ) ) ;
#5297=CARTESIAN_POINT ( 'NONE',  ( -31.00000000000000711, -15.00000000000000000, 6.000000000000009770 ) ) ;
#5315=CARTESIAN_POINT ( 'NONE',  ( -0.9115637956585259660, -11.70315718320097886, 38.99939858132674431 ) ) ;
#5326=LINE ( 'NONE', #3638, #2618 ) ;
#5330=FACE_OUTER_BOUND ( 'NONE', #9136, .T. ) ;
#5332=CARTESIAN_POINT ( 'NONE',  ( -10.00000000000001599, 3.294852476658805873, 41.36423575989289247 ) ) ;
#5333=ORIENTED_EDGE ( 'NONE', *, *, #9565, .T. ) ;
#5335=CARTESIAN_POINT ( 'NONE',  ( 5.824897344823916079, -8.145636269817515540, 38.91941837930603754 ) ) ;
#5339=CARTESIAN_POINT ( 'NONE',  ( 0.000000000000000000, 3.294852476641296768, 184.6745183374407020 ) ) ;
#5341=CARTESIAN_POINT ( 'NONE',  ( 9.998295632719816695, 2.529332002499826704, 37.85922636131657271 ) ) ;
#5345=DIRECTION ( 'NONE',  ( 0.07726494571055114724, 0.000000000000000000, 0.9970105958134776181 ) ) ;
#5362=CARTESIAN_POINT ( 'NONE',  ( 0.000000000000000000, 3.294852476641296768, 294.6136752714472777 ) ) ;
#5366=VECTOR ( 'NONE', #422, 1000.000000000000000 ) ;
#5372=CARTESIAN_POINT ( 'NONE',  ( 1.314778108344340835, -6.640250172933917838, 43.96652902435248933 ) ) ;
#5385=CARTESIAN_POINT ( 'NONE',  ( 1.066084653997754650, -14.99999999999968203, 36.76550911089076124 ) ) ;
#5389=CARTESIAN_POINT ( 'NONE',  ( -6.000000000000005329, 29.14236109046821710, -29.24912810952613640 ) ) ;
#5390=ORIENTED_EDGE ( 'NONE', *, *, #6063, .F. ) ;
#5391=CARTESIAN_POINT ( 'NONE',  ( 9.872059229381315859, 4.922636072021620457, 41.43345053423059454 ) ) ;
#5396=DIRECTION ( 'NONE',  ( -1.000000000000000000, 0.000000000000000000, 0.000000000000000000 ) ) ;
#5414=( NAMED_UNIT ( * ) PLANE_ANGLE_UNIT ( ) SI_UNIT ( $, .RADIAN. ) );
#5424=CARTESIAN_POINT ( 'NONE',  ( 2.604746439356475207, -6.365628610964990663, 43.82878309350103763 ) ) ;
#5429=CARTESIAN_POINT ( 'NONE',  ( -31.00000000000001066, 27.61361909880193011, 5.005767756411737324 ) ) ;
#5433=LINE ( 'NONE', #2597, #6400 ) ;
#5434=ORIENTED_EDGE ( 'NONE', *, *, #761, .T. ) ;
#5436=DIRECTION ( 'NONE',  ( -0.000000000000000000, 1.000000000000000000, -0.000000000000000000 ) ) ;
#5441=CARTESIAN_POINT ( 'NONE',  ( 4.433825966365425586, -5.692418513649885270, 43.50410792870121668 ) ) ;
#5447=ORIENTED_EDGE ( 'NONE', *, *, #93, .F. ) ;
#5455=ORIENTED_EDGE ( 'NONE', *, *, #8532, .T. ) ;
#5463=CARTESIAN_POINT ( 'NONE',  ( -5.042085649091919919, -5.365591822504794273, 43.35300965850710497 ) ) ;
#5473=EDGE_CURVE ( 'NONE', #8960, #1381, #3383, .T. ) ;
#5482=ADVANCED_FACE ( 'NONE', ( #6771 ), #6899, .F. ) ;
#5487=DIRECTION ( 'NONE',  ( 0.000000000000000000, -1.000000000000000000, 0.000000000000000000 ) ) ;
#5491=CARTESIAN_POINT ( 'NONE',  ( 0.000000000000000000, -15.00000000000000000, 0.000000000000000000 ) ) ;
#5494=CARTESIAN_POINT ( 'NONE',  ( -31.00000000000000711, -15.00000000000000000, -5.999999999999996447 ) ) ;
#5497=CARTESIAN_POINT ( 'NONE',  ( 8.237197373723128990, -4.999999999999999112, 27.80554943579302574 ) ) ;
#5498=CARTESIAN_POINT ( 'NONE',  ( -5.999999999999998224, -15.00000000000000000, 26.32489316217636954 ) ) ;
#5502=EDGE_CURVE ( 'NONE', #6350, #7928, #8339, .T. ) ;
#5503=CARTESIAN_POINT ( 'NONE',  ( -2.637864787425444835, -6.356637827719301193, 43.82432124711748855 ) ) ;
#5506=VERTEX_POINT ( 'NONE', #7619 ) ;
#5509=CARTESIAN_POINT ( 'NONE',  ( -6.323936101127149989, -4.493502404820619134, 38.59188261056448965 ) ) ;
#5515=CARTESIAN_POINT ( 'NONE',  ( 4.776122516674680244E-15, 19.99999999999982236, 39.00000000000002132 ) ) ;
#5519=LINE ( 'NONE', #7643, #7800 ) ;
#5522=EDGE_CURVE ( 'NONE', #6324, #2298, #4336, .T. ) ;
#5535=CARTESIAN_POINT ( 'NONE',  ( 8.758195361064911921, -8.001464458227651733, 38.00543791605778665 ) ) ;
#5540=ORIENTED_EDGE ( 'NONE', *, *, #3736, .F. ) ;
#5545=AXIS2_PLACEMENT_3D ( 'NONE', #6194, #3276, #2579 ) ;
#5552=CARTESIAN_POINT ( 'NONE',  ( -12.59566441936335757, -1.532720036839458899, 36.91025998118985996 ) ) ;
#5553=CARTESIAN_POINT ( 'NONE',  ( 0.000000000000000000, 30.00000000000000000, 0.000000000000000000 ) ) ;
#5556=ORIENTED_EDGE ( 'NONE', *, *, #6366, .F. ) ;
#5558=EDGE_LOOP ( 'NONE', ( #7451, #1099, #8769, #3445 ) ) ;
#5600=CARTESIAN_POINT ( 'NONE',  ( -8.684397385907152156, -1.706296020601628216, 42.03131819750302611 ) ) ;
#5614=LINE ( 'NONE', #2483, #8981 ) ;
#5615=CARTESIAN_POINT ( 'NONE',  ( 11.24085533630444544, -4.722505971463051289, 37.34530973190163650 ) ) ;
#5624=B_SPLINE_CURVE_WITH_KNOTS ( 'NONE', 3,
 ( #2988, #2186, #5954, #5997 ),
 .UNSPECIFIED., .F., .F.,
 ( 4, 4 ),
 ( 8.673617379884035472E-19, 0.006018989108141225772 ),
 .UNSPECIFIED. ) ;
#5633=CARTESIAN_POINT ( 'NONE',  ( 8.083702140090636590, -8.624291467721789672, 38.15459417795183583 ) ) ;
#5634=ORIENTED_EDGE ( 'NONE', *, *, #5502, .T. ) ;
#5653=CARTESIAN_POINT ( 'NONE',  ( -5.536480372579049458, -5.071221366488331661, 38.69702195666404521 ) ) ;
#5658=ORIENTED_EDGE ( 'NONE', *, *, #8395, .F. ) ;
#5664=CARTESIAN_POINT ( 'NONE',  ( 12.40150588385810515, 8.712168704539934083, 36.97588844760274895 ) ) ;
#5668=EDGE_LOOP ( 'NONE', ( #7409, #4714, #8742, #8283, #2494 ) ) ;
#5671=ORIENTED_EDGE ( 'NONE', *, *, #6544, .T. ) ;
#5672=DIRECTION ( 'NONE',  ( 0.000000000000000000, -0.000000000000000000, -1.000000000000000000 ) ) ;
#5675=LINE ( 'NONE', #3250, #7776 ) ;
#5682=CARTESIAN_POINT ( 'NONE',  ( -7.625823958607668374, -7.198980154853257929, 38.46531392912545755 ) ) ;
#5687=CARTESIAN_POINT ( 'NONE',  ( 2.632839041009112258, 12.96455383109111814, 43.83318083222629014 ) ) ;
#5693=ORIENTED_EDGE ( 'NONE', *, *, #8313, .T. ) ;
#5696=CARTESIAN_POINT ( 'NONE',  ( -7.754730899493599061, -3.063035541202936418, 38.35473839958616793 ) ) ;
#5705=EDGE_CURVE ( 'NONE', #7606, #874, #6993, .T. ) ;
#5708=FACE_OUTER_BOUND ( 'NONE', #9529, .T. ) ;
#5710=EDGE_CURVE ( 'NONE', #1760, #6269, #7849, .T. ) ;
#5711=DIRECTION ( 'NONE',  ( -0.000000000000000000, -0.000000000000000000, 1.000000000000000000 ) ) ;
#5713=ORIENTED_EDGE ( 'NONE', *, *, #868, .T. ) ;
#5723=AXIS2_PLACEMENT_3D ( 'NONE', #5059, #8861, #9747 ) ;
#5728=CARTESIAN_POINT ( 'NONE',  ( -2.808770322584149604, -15.00000000000000000, 29.89902100188472645 ) ) ;
#5733=CARTESIAN_POINT ( 'NONE',  ( 5.037425304447057606, 11.93964564789587790, 43.34856681498735043 ) ) ;
#5734=ORIENTED_EDGE ( 'NONE', *, *, #5757, .T. ) ;
#5739=ADVANCED_FACE ( 'NONE', ( #5998 ), #4338, .T. ) ;
#5741=CARTESIAN_POINT ( 'NONE',  ( 0.01843853347452210911, 13.29483547765103069, 43.99999130734106245 ) ) ;
#5742=VECTOR ( 'NONE', #6626, 1000.000000000000000 ) ;
#5749=ORIENTED_EDGE ( 'NONE', *, *, #5502, .F. ) ;
#5755=EDGE_CURVE ( 'NONE', #9184, #1828, #8979, .T. ) ;
#5757=EDGE_CURVE ( 'NONE', #4378, #1718, #2188, .T. ) ;
#5758=CARTESIAN_POINT ( 'NONE',  ( 0.000000000000000000, 30.00000000000000000, 0.000000000000000000 ) ) ;
#5759=AXIS2_PLACEMENT_3D ( 'NONE', #5297, #855, #8309 ) ;
#5761=AXIS2_PLACEMENT_3D ( 'NONE', #6524, #8020, #5058 ) ;
#5764=PLANE ( 'NONE',  #4226 ) ;
#5765=CARTESIAN_POINT ( 'NONE',  ( 10.00000000000001599, 3.294852476638864491, 41.36423575989288537 ) ) ;
#5768=EDGE_LOOP ( 'NONE', ( #4276, #2840, #2759, #3698, #2971, #8896, #513, #3030, #5969, #2136, #4072, #7470, #4223, #2814, #3466, #134 ) ) ;
#5774=CARTESIAN_POINT ( 'NONE',  ( -6.000000000000005329, -10.00000000000000533, -26.32489316217636954 ) ) ;
#5783=CARTESIAN_POINT ( 'NONE',  ( -8.329014317829159353, -6.778170143341801790, 38.25993911327689290 ) ) ;
#5788=CARTESIAN_POINT ( 'NONE',  ( 3.885102854800722483, 12.53650132828193797, 38.86177049418535034 ) ) ;
#5796=CARTESIAN_POINT ( 'NONE',  ( -8.116472182054980777, 9.145332620307328853, 42.28305399575716450 ) ) ;
#5797=EDGE_CURVE ( 'NONE', #1718, #9349, #7487, .T. ) ;
#5801=CARTESIAN_POINT ( 'NONE',  ( 31.00000000000000711, -15.00000000000000000, 6.000000000000000000 ) ) ;
#5804=CARTESIAN_POINT ( 'NONE',  ( 31.00000000000000711, 27.42469319230601243, 6.000000000000000000 ) ) ;
#5805=CARTESIAN_POINT ( 'NONE',  ( -31.00000000000000711, 27.42469319230601243, -5.999999999999996447 ) ) ;
#5806=CARTESIAN_POINT ( 'NONE',  ( 12.50302036141013140, 8.406344128993804787, 36.94162958640247751 ) ) ;
#5809=ADVANCED_FACE ( 'NONE', ( #8089 ), #4396, .T. ) ;
#5813=CARTESIAN_POINT ( 'NONE',  ( 10.00000000000009948, 3.626867479774634084, 41.36423575989284274 ) ) ;
#5816=CARTESIAN_POINT ( 'NONE',  ( -13.15959852261851815, 1.059259259969981937, 36.71292293559446307 ) ) ;
#5822=CARTESIAN_POINT ( 'NONE',  ( -0.4572298495115817429, -15.00000000000015987, 36.76400391796496336 ) ) ;
#5823=ORIENTED_EDGE ( 'NONE', *, *, #166, .T. ) ;
#5824=EDGE_CURVE ( 'NONE', #9481, #2330, #3104, .T. ) ;
#5831=CARTESIAN_POINT ( 'NONE',  ( 10.01906723522320064, 13.16737651941478049, 37.69215544616801594 ) ) ;
#5857=CARTESIAN_POINT ( 'NONE',  ( 5.326140061663600100, 11.76457241320986924, 43.27053568042958887 ) ) ;
#5865=CARTESIAN_POINT ( 'NONE',  ( -3.910602396084473575, -8.894839577748838266, 39.26794276223228053 ) ) ;
#5866=AXIS2_PLACEMENT_3D ( 'NONE', #985, #4844, #6408 ) ;
#5870=ORIENTED_EDGE ( 'NONE', *, *, #3455, .T. ) ;
#5873=CARTESIAN_POINT ( 'NONE',  ( 4.720363748491940292, 12.14410912167428869, 38.78759026100516394 ) ) ;
#5874=EDGE_CURVE ( 'NONE', #5016, #2330, #5519, .T. ) ;
#5883=CARTESIAN_POINT ( 'NONE',  ( -9.686515203225052772, 13.58116064233279552, 37.77923906255211506 ) ) ;
#5890=ORIENTED_EDGE ( 'NONE', *, *, #9744, .F. ) ;
#5903=CARTESIAN_POINT ( 'NONE',  ( 1.773930110362821555, -15.00000000000000178, 30.27515255412638240 ) ) ;
#5905=CARTESIAN_POINT ( 'NONE',  ( -4.424613605680260520, 17.45796735942974109, 38.75301155415253618 ) ) ;
#5915=CARTESIAN_POINT ( 'NONE',  ( 10.67347934733978754, -5.256592221152843969, 37.51339085603135004 ) ) ;
#5922=CARTESIAN_POINT ( 'NONE',  ( 9.601051617431352270, 6.203770162293365864, 37.95839508490225711 ) ) ;
#5923=SHAPE_DEFINITION_REPRESENTATION ( #4738, #5213 ) ;
#5932=EDGE_LOOP ( 'NONE', ( #9186, #8422, #2875, #4161, #3647, #6278, #5264 ) ) ;
#5933=CARTESIAN_POINT ( 'NONE',  ( -1.294388769339064327, 13.21620364998245023, 43.95989878156864705 ) ) ;
#5938=VERTEX_POINT ( 'NONE', #9133 ) ;
#5951=CARTESIAN_POINT ( 'NONE',  ( 7.522530930366955637, -3.325240747455041834, 42.53435141087333449 ) ) ;
#5954=CARTESIAN_POINT ( 'NONE',  ( 2.008133409164431615, 27.99999999999992184, -31.00000000000000711 ) ) ;
#5955=CARTESIAN_POINT ( 'NONE',  ( 0.000000000000000000, -4.999999999999999112, 0.000000000000000000 ) ) ;
#5959=CARTESIAN_POINT ( 'NONE',  ( 10.60693692882557038, -15.00000000000062528, 37.26904593215826367 ) ) ;
#5964=CARTESIAN_POINT ( 'NONE',  ( 9.114420836480412902, 7.422247012081075290, 41.82255323698446148 ) ) ;
#5969=ORIENTED_EDGE ( 'NONE', *, *, #197, .F. ) ;
#5974=DIRECTION ( 'NONE',  ( 0.000000000000000000, 0.000000000000000000, -1.000000000000000000 ) ) ;
#5975=B_SPLINE_CURVE_WITH_KNOTS ( 'NONE', 3,
 ( #3226, #9019, #6036, #875 ),
 .UNSPECIFIED., .F., .F.,
 ( 4, 4 ),
 ( 8.673617379884035472E-19, 0.006018989108141226639 ),
 .UNSPECIFIED. ) ;
#5977=AXIS2_PLACEMENT_3D ( 'NONE', #1798, #4825, #1064 ) ;
#5978=EDGE_LOOP ( 'NONE', ( #306, #8745, #993, #5658 ) ) ;
#5981=ORIENTED_EDGE ( 'NONE', *, *, #1724, .F. ) ;
#5983=CARTESIAN_POINT ( 'NONE',  ( 0.000000000000000000, -15.00000000000000000, 0.000000000000000000 ) ) ;
#5988=CARTESIAN_POINT ( 'NONE',  ( 2.040301830986985809, -9.344775919449732626, 39.47202367093716191 ) ) ;
#5996=CARTESIAN_POINT ( 'NONE',  ( 0.3582566269629631206, -15.00000000000000000, 30.57108970959263416 ) ) ;
#5997=CARTESIAN_POINT ( 'NONE',  ( 1.221566888952841201E-22, 27.99999999999992184, -31.00000000000000711 ) ) ;
#5998=FACE_OUTER_BOUND ( 'NONE', #5978, .T. ) ;
#5999=EDGE_CURVE ( 'NONE', #6799, #4378, #8596, .T. ) ;
#6004=CARTESIAN_POINT ( 'NONE',  ( 4.909944792989705320, -8.520966008424666782, 39.09496844136518945 ) ) ;
#6011=CARTESIAN_POINT ( 'NONE',  ( 8.648354992365815619, -1.736301028422764903, 42.04488899069198027 ) ) ;
#6017=FACE_OUTER_BOUND ( 'NONE', #4144, .T. ) ;
#6034=CARTESIAN_POINT ( 'NONE',  ( 4.035851918958802464, -8.834948306663564566, 39.24029717320215127 ) ) ;
#6036=CARTESIAN_POINT ( 'NONE',  ( -2.008133409164426730, 27.99999999999992184, 31.00000000000000711 ) ) ;
#6039=CARTESIAN_POINT ( 'NONE',  ( 6.105199365910152665, -4.651526790810022405, 43.04426269254581428 ) ) ;
#6046=EDGE_CURVE ( 'NONE', #2330, #1923, #8540, .T. ) ;
#6056=CARTESIAN_POINT ( 'NONE',  ( 6.933488530059848109, -15.00000000000000000, 36.84292232056203886 ) ) ;
#6061=ADVANCED_FACE ( 'NONE', ( #2586 ), #9238, .T. ) ;
#6063=EDGE_CURVE ( 'NONE', #4609, #9521, #4239, .T. ) ;
#6064=DIRECTION ( 'NONE',  ( -0.000000000000000000, -0.000000000000000000, 1.000000000000000000 ) ) ;
#6067=AXIS2_PLACEMENT_3D ( 'NONE', #3654, #8892, #8989 ) ;
#6069=CARTESIAN_POINT ( 'NONE',  ( 9.737083392141938631, 0.9931181127733758052, 41.50525870069961343 ) ) ;
#6071=STYLED_ITEM('',(#9771),#6323);
#6079=AXIS2_PLACEMENT_3D ( 'NONE', #5339, #6064, #848 ) ;
#6083=CARTESIAN_POINT ( 'NONE',  ( -6.858200383473443296, -3.989910541781668485, 42.78193147746105751 ) ) ;
#6084=VECTOR ( 'NONE', #1119, 1000.000000000000000 ) ;
#6092=CARTESIAN_POINT ( 'NONE',  ( -5.942969066593652094, -10.15910374927029736, 38.55304109327786222 ) ) ;
#6096=ORIENTED_EDGE ( 'NONE', *, *, #521, .T. ) ;
#6099=ORIENTED_EDGE ( 'NONE', *, *, #9562, .T. ) ;
#6100=CARTESIAN_POINT ( 'NONE',  ( 7.931830219867401333, -2.829627378531556658, 42.36468407235587819 ) ) ;
#6102=CARTESIAN_POINT ( 'NONE',  ( 3.475261766519177176, -15.00000000000000178, 29.62668451659027014 ) ) ;
#6104=ORIENTED_EDGE ( 'NONE', *, *, #9328, .T. ) ;
#6110=CARTESIAN_POINT ( 'NONE',  ( 5.540660272217056814, -15.00000000000031619, 36.79964862145148174 ) ) ;
#6115=VERTEX_POINT ( 'NONE', #8579 ) ;
#6116=CARTESIAN_POINT ( 'NONE',  ( 12.83676879653350866, -0.6422030776960447884, 36.82710757287565428 ) ) ;
#6120=PLANE ( 'NONE',  #2498 ) ;
#6129=CARTESIAN_POINT ( 'NONE',  ( -6.123066174590870325, -4.617945597878252428, 43.03242323456579754 ) ) ;
#6137=VECTOR ( 'NONE', #5345, 1000.000000000000000 ) ;
#6141=CARTESIAN_POINT ( 'NONE',  ( 31.00000000000000711, -15.00000000000000000, 6.000000000000000000 ) ) ;
#6146=CARTESIAN_POINT ( 'NONE',  ( -8.237197373723139648, -15.00000000000000000, 27.80554943579302929 ) ) ;
#6161=CARTESIAN_POINT ( 'NONE',  ( -6.000000000000005329, 27.42469319230600533, -31.00000000000000711 ) ) ;
#6163=CARTESIAN_POINT ( 'NONE',  ( 6.290056143031378610, -4.520955051545493042, 38.59677555533873772 ) ) ;
#6170=ORIENTED_EDGE ( 'NONE', *, *, #6662, .F. ) ;
#6176=EDGE_CURVE ( 'NONE', #3412, #8756, #8870, .T. ) ;
#6180=ORIENTED_EDGE ( 'NONE', *, *, #8964, .T. ) ;
#6182=CARTESIAN_POINT ( 'NONE',  ( -4.469925451758544277, -5.674451673807808127, 43.49573866965157976 ) ) ;
#6194=CARTESIAN_POINT ( 'NONE',  ( 0.000000000000000000, 19.99999999999982236, 0.000000000000000000 ) ) ;
#6197=CARTESIAN_POINT ( 'NONE',  ( 6.168569856766713322, 16.58737218350495723, 38.51007260663249099 ) ) ;
#6221=CARTESIAN_POINT ( 'NONE',  ( -6.620899530561116464, -4.206347570868084418, 42.86624096190644906 ) ) ;
#6223=VECTOR ( 'NONE', #4189, 1000.000000000000000 ) ;
#6227=CIRCLE ( 'NONE', #3394, 28.99999999999995026 ) ;
#6235=( GEOMETRIC_REPRESENTATION_CONTEXT ( 3 ) GLOBAL_UNCERTAINTY_ASSIGNED_CONTEXT ( ( #814 ) ) GLOBAL_UNIT_ASSIGNED_CONTEXT ( ( #3122, #5414, #6921 ) ) REPRESENTATION_CONTEXT ( 'NONE', 'WORKASPACE' ) );
#6236=CARTESIAN_POINT ( 'NONE',  ( -9.920757921939857837, 1.831472460275451519, 37.87927513041881866 ) ) ;
#6238=CARTESIAN_POINT ( 'NONE',  ( 0.01843853345419280837, 13.29483547765106799, 43.99999130734108377 ) ) ;
#6262=CARTESIAN_POINT ( 'NONE',  ( 0.6466180781814862000, -6.706436388010658334, 44.00065907709070245 ) ) ;
#6265=ORIENTED_EDGE ( 'NONE', *, *, #3689, .T. ) ;
#6269=VERTEX_POINT ( 'NONE', #6728 ) ;
#6277=ORIENTED_EDGE ( 'NONE', *, *, #9704, .F. ) ;
#6278=ORIENTED_EDGE ( 'NONE', *, *, #8114, .F. ) ;
#6279=CARTESIAN_POINT ( 'NONE',  ( -13.27241307482885802, 4.308278809869828585, 36.67213216020381594 ) ) ;
#6280=DIRECTION ( 'NONE',  ( -0.000000000000000000, 1.000000000000000000, -0.000000000000000000 ) ) ;
#6283=DIRECTION ( 'NONE',  ( 0.000000000000000000, 0.000000000000000000, -1.000000000000000000 ) ) ;
#6291=CIRCLE ( 'NONE', #8189, 39.00000000000002132 ) ;
#6293=EDGE_CURVE ( 'NONE', #1923, #5073, #5132, .T. ) ;
#6296=DIRECTION ( 'NONE',  ( -0.001843853345419366619, -0.9999983001009754568, 0.000000000000000000 ) ) ;
#6302=DIRECTION ( 'NONE',  ( 0.000000000000000000, -1.000000000000000000, 0.000000000000000000 ) ) ;
#6303=CARTESIAN_POINT ( 'NONE',  ( 10.00000000000001599, 3.294852476641296768, 184.6745183374407020 ) ) ;
#6305=CARTESIAN_POINT ( 'NONE',  ( -9.669395431759557624, 5.928981332583603603, 41.54124299433283340 ) ) ;
#6311=EDGE_CURVE ( 'NONE', #285, #8477, #888, .T. ) ;
#6314=AXIS2_PLACEMENT_3D ( 'NONE', #9654, #2830, #5168 ) ;
#6317=ORIENTED_EDGE ( 'NONE', *, *, #9704, .T. ) ;
#6319=ORIENTED_EDGE ( 'NONE', *, *, #9328, .F. ) ;
#6323=MANIFOLD_SOLID_BREP ( 'Chamfer5', #3571 ) ;
#6324=VERTEX_POINT ( 'NONE', #6238 ) ;
#6329=ORIENTED_EDGE ( 'NONE', *, *, #7081, .T. ) ;
#6330=CARTESIAN_POINT ( 'NONE',  ( -9.866411883523234394, 4.956617588930513740, 41.43648181959947152 ) ) ;
#6340=AXIS2_PLACEMENT_3D ( 'NONE', #9730, #4549, #743 ) ;
#6347=AXIS2_PLACEMENT_3D ( 'NONE', #7041, #5487, #4789 ) ;
#6350=VERTEX_POINT ( 'NONE', #3776 ) ;
#6363=DIRECTION ( 'NONE',  ( -0.9588120495101037921, 0.000000000000000000, 0.2840412887490734173 ) ) ;
#6364=CARTESIAN_POINT ( 'NONE',  ( 3.796404955196288922E-15, 27.99999999999992184, 31.00000000000000711 ) ) ;
#6366=EDGE_CURVE ( 'NONE', #7266, #2358, #2921, .T. ) ;
#6371=AXIS2_PLACEMENT_3D ( 'NONE', #4984, #549, #8692 ) ;
#6379=ORIENTED_EDGE ( 'NONE', *, *, #6477, .F. ) ;
#6380=CARTESIAN_POINT ( 'NONE',  ( -9.350470702154407121, 6.934942045775910557, 38.01926452046366478 ) ) ;
#6385=VECTOR ( 'NONE', #4846, 1000.000000000000000 ) ;
#6393=CYLINDRICAL_SURFACE ( 'NONE', #1103, 27.00000000000000355 ) ;
#6395=PLANE ( 'NONE',  #1420 ) ;
#6396=DIRECTION ( 'NONE',  ( 1.000000000000000000, 0.000000000000000000, 0.000000000000000000 ) ) ;
#6400=VECTOR ( 'NONE', #897, 1000.000000000000000 ) ;
#6403=CARTESIAN_POINT ( 'NONE',  ( 6.622760353406874856, 10.81530383135506135, 42.86969992518040584 ) ) ;
#6405=CARTESIAN_POINT ( 'NONE',  ( 0.000000000000000000, 19.99999999999982236, 0.000000000000000000 ) ) ;
#6408=DIRECTION ( 'NONE',  ( 0.000000000000000000, 0.000000000000000000, -1.000000000000000000 ) ) ;
#6414=CARTESIAN_POINT ( 'NONE',  ( -10.60768798165303473, -14.99999999999749356, 37.26924479348801356 ) ) ;
#6418=CARTESIAN_POINT ( 'NONE',  ( 0.4611600587751271130, 18.29391864775294962, 38.99971782587474678 ) ) ;
#6429=CARTESIAN_POINT ( 'NONE',  ( -12.84969364742680753, -0.5881807229699745898, 36.82259397722437910 ) ) ;
#6437=DIRECTION ( 'NONE',  ( -1.000000000000000000, 0.000000000000000000, 0.000000000000000000 ) ) ;
#6438=CARTESIAN_POINT ( 'NONE',  ( 6.981204600336408994, 16.06533569283885399, 38.37097370016179809 ) ) ;
#6440=DIRECTION ( 'NONE',  ( 0.000000000000000000, 0.000000000000000000, -1.000000000000000000 ) ) ;
#6441=B_SPLINE_CURVE_WITH_KNOTS ( 'NONE', 3,
 ( #3157, #14, #9106, #3008 ),
 .UNSPECIFIED., .F., .F.,
 ( 4, 4 ),
 ( 9.813077866773594792E-18, 0.003679109433542027217 ),
 .UNSPECIFIED. ) ;
#6443=CARTESIAN_POINT ( 'NONE',  ( -10.00000000000001599, 3.294852476641298100, 184.6745183374407020 ) ) ;
#6456=CARTESIAN_POINT ( 'NONE',  ( -1.435128562976363265, -14.99999999999999822, 30.37910621253763566 ) ) ;
#6461=CARTESIAN_POINT ( 'NONE',  ( 2.216463206349838178, 13.07088745734695934, 38.96084410410938403 ) ) ;
#6466=ORIENTED_EDGE ( 'NONE', *, *, #4794, .T. ) ;
#6475=EDGE_CURVE ( 'NONE', #2998, #4074, #3552, .T. ) ;
#6477=EDGE_CURVE ( 'NONE', #6561, #1456, #283, .T. ) ;
#6479=CARTESIAN_POINT ( 'NONE',  ( -10.23819876369190318, -5.532962098992985744, 37.64233965054218345 ) ) ;
#6482=EDGE_LOOP ( 'NONE', ( #2868, #2159, #6697, #8247, #4701 ) ) ;
#6496=CARTESIAN_POINT ( 'NONE',  ( 7.525660590371140657, 9.887872461981832117, 42.52846908860392716 ) ) ;
#6503=AXIS2_PLACEMENT_3D ( 'NONE', #4447, #112, #3749 ) ;
#6504=CARTESIAN_POINT ( 'NONE',  ( 8.982437128886548550, -6.367019354910812723, 38.05793569061005144 ) ) ;
#6511=CARTESIAN_POINT ( 'NONE',  ( -7.751339229931619279, -15.00000000000000355, 36.88905299132577653 ) ) ;
#6515=CARTESIAN_POINT ( 'NONE',  ( -5.999999999999998224, -15.00000000000000000, 31.00000000000000711 ) ) ;
#6516=CARTESIAN_POINT ( 'NONE',  ( 0.02451486834250751756, 18.29482697815594605, 38.99999229514322963 ) ) ;
#6522=ORIENTED_EDGE ( 'NONE', *, *, #166, .F. ) ;
#6523=CARTESIAN_POINT ( 'NONE',  ( 0.01529561596030615950, 13.29484127273986260, 38.99999809024075148 ) ) ;
#6524=CARTESIAN_POINT ( 'NONE',  ( 0.000000000000000000, -4.999999999999997335, 0.000000000000000000 ) ) ;
#6527=AXIS2_PLACEMENT_3D ( 'NONE', #5079, #7399, #8188 ) ;
#6531=EDGE_CURVE ( 'NONE', #6561, #1760, #9085, .T. ) ;
#6534=AXIS2_PLACEMENT_3D ( 'NONE', #5497, #6363, #4162 ) ;
#6537=CARTESIAN_POINT ( 'NONE',  ( 9.145707437616094282, 14.18749288135022368, 37.91311953629105602 ) ) ;
#6544=EDGE_CURVE ( 'NONE', #2358, #7266, #1671, .T. ) ;
#6547=FACE_OUTER_BOUND ( 'NONE', #932, .T. ) ;
#6551=ORIENTED_EDGE ( 'NONE', *, *, #8609, .T. ) ;
#6554=VECTOR ( 'NONE', #8306, 1000.000000000000000 ) ;
#6561=VERTEX_POINT ( 'NONE', #1257 ) ;
#6563=CARTESIAN_POINT ( 'NONE',  ( -2.136419886453954309, -9.299694386856355521, 39.45120225348325960 ) ) ;
#6568=CARTESIAN_POINT ( 'NONE',  ( 8.807406495666141311, 14.57426945197969381, 37.99774521171899977 ) ) ;
#6577=CARTESIAN_POINT ( 'NONE',  ( -9.479506463030828556, 6.546681192253595682, 41.64102178833953616 ) ) ;
#6581=DIRECTION ( 'NONE',  ( -0.000000000000000000, 1.000000000000000000, -0.000000000000000000 ) ) ;
#6586=DIRECTION ( 'NONE',  ( -0.000000000000000000, -0.000000000000000000, 1.000000000000000000 ) ) ;
#6592=CARTESIAN_POINT ( 'NONE',  ( 1.675417577077328968, 13.15907318124163616, 43.93088470327393225 ) ) ;
#6595=CARTESIAN_POINT ( 'NONE',  ( -5.999999999999998224, 27.42469319230601243, 31.00000000000000711 ) ) ;
#6599=DIRECTION ( 'NONE',  ( 0.000000000000000000, 0.000000000000000000, 1.000000000000000000 ) ) ;
#6601=CARTESIAN_POINT ( 'NONE',  ( 0.02042900839392215728, 18.29483547775932095, 38.99999486345961941 ) ) ;
#6602=CARTESIAN_POINT ( 'NONE',  ( -7.537816291435827765, -14.99999999999999822, 28.01273613541154361 ) ) ;
#6604=ADVANCED_FACE ( 'NONE', ( #3668 ), #4318, .T. ) ;
#6618=LINE ( 'NONE', #8632, #6084 ) ;
#6621=CARTESIAN_POINT ( 'NONE',  ( -11.51340233387757017, 10.85928029369878267, 37.26517847978107767 ) ) ;
#6626=DIRECTION ( 'NONE',  ( 0.000000000000000000, 0.000000000000000000, 1.000000000000000000 ) ) ;
#6640=CARTESIAN_POINT ( 'NONE',  ( -31.00000000000000355, 27.99909559099847911, -2.017392264862527096 ) ) ;
#6647=CARTESIAN_POINT ( 'NONE',  ( 8.323710113664041899, -6.781460580756969669, 38.26155278793961401 ) ) ;
#6655=CARTESIAN_POINT ( 'NONE',  ( 8.908588037261978343, 7.879430400622490005, 38.11900311772433270 ) ) ;
#6662=EDGE_CURVE ( 'NONE', #7666, #6561, #7828, .T. ) ;
#6667=CARTESIAN_POINT ( 'NONE',  ( -2.597462001549401212, 12.97425228067757175, 43.83800940528956858 ) ) ;
#6669=CARTESIAN_POINT ( 'NONE',  ( -6.000000000000005329, 27.42469319230600533, -31.00000000000000711 ) ) ;
#6670=ORIENTED_EDGE ( 'NONE', *, *, #1180, .F. ) ;
#6674=DIRECTION ( 'NONE',  ( 0.000000000000000000, -0.000000000000000000, -1.000000000000000000 ) ) ;
#6682=DIRECTION ( 'NONE',  ( 0.000000000000000000, 0.000000000000000000, -1.000000000000000000 ) ) ;
#6685=CARTESIAN_POINT ( 'NONE',  ( 4.817158075008645568, -15.00000000000000178, 29.05778733718146611 ) ) ;
#6686=CARTESIAN_POINT ( 'NONE',  ( 30.12488991936162108, 28.28385863652523824, -6.000000000000006217 ) ) ;
#6687=CARTESIAN_POINT ( 'NONE',  ( -2.254158640986140050, 18.08224550467000569, 38.93613429042778051 ) ) ;
#6691=VECTOR ( 'NONE', #8154, 1000.000000000000000 ) ;
#6697=ORIENTED_EDGE ( 'NONE', *, *, #9513, .F. ) ;
#6699=CARTESIAN_POINT ( 'NONE',  ( 7.536687028107835751, -15.00000000000000000, 28.01307067288326280 ) ) ;
#6706=CARTESIAN_POINT ( 'NONE',  ( 11.91013294755531149, -3.389816855901808701, 37.13751894432687806 ) ) ;
#6708=ORIENTED_EDGE ( 'NONE', *, *, #1792, .F. ) ;
#6725=CARTESIAN_POINT ( 'NONE',  ( -5.044664205793679024, -8.473593863896581979, 39.07304412537308025 ) ) ;
#6728=CARTESIAN_POINT ( 'NONE',  ( 6.439978105601112524E-15, 18.29485247664131009, 39.00000000000002132 ) ) ;
#6733=CARTESIAN_POINT ( 'NONE',  ( 0.000000000000000000, 19.99999999999982236, 0.000000000000000000 ) ) ;
#6734=DIRECTION ( 'NONE',  ( 0.000000000000000000, 0.000000000000000000, -1.000000000000000000 ) ) ;
#6738=CARTESIAN_POINT ( 'NONE',  ( -2.575401375589585040, 18.01522921748959405, 38.91614804012162665 ) ) ;
#6744=CARTESIAN_POINT ( 'NONE',  ( 0.8972019483868172163, -15.00000000000000000, 30.49724507882217495 ) ) ;
#6747=CARTESIAN_POINT ( 'NONE',  ( 0.000000000000000000, 3.294852476641296768, 184.6745183374407020 ) ) ;
#6749=CARTESIAN_POINT ( 'NONE',  ( 9.098375990985465123, -0.8675798692180576310, 41.83041446991980905 ) ) ;
#6754=ORIENTED_EDGE ( 'NONE', *, *, #4265, .T. ) ;
#6761=CARTESIAN_POINT ( 'NONE',  ( -2.318347576506052388, -6.438274054832179516, 43.86504657511039085 ) ) ;
#6770=FACE_OUTER_BOUND ( 'NONE', #3365, .T. ) ;
#6771=FACE_OUTER_BOUND ( 'NONE', #5932, .T. ) ;
#6792=CARTESIAN_POINT ( 'NONE',  ( -31.00000000000000711, 30.00000000000000000, -5.999999999999996447 ) ) ;
#6798=CARTESIAN_POINT ( 'NONE',  ( 7.229529499415464855, -7.426880451839177333, 38.57586176292668512 ) ) ;
#6799=VERTEX_POINT ( 'NONE', #9056 ) ;
#6800=AXIS2_PLACEMENT_3D ( 'NONE', #7869, #7006, #1874 ) ;
#6805=CARTESIAN_POINT ( 'NONE',  ( 9.920401881134884192, 4.597042934328839259, 41.40737016411131322 ) ) ;
#6808=ORIENTED_EDGE ( 'NONE', *, *, #7755, .T. ) ;
#6815=CARTESIAN_POINT ( 'NONE',  ( -1.639856434810980312, 13.16510872014126221, 43.93393704144139633 ) ) ;
#6818=DIRECTION ( 'NONE',  ( 1.000000000000000000, 0.000000000000000000, 0.000000000000000000 ) ) ;
#6819=AXIS2_PLACEMENT_3D ( 'NONE', #7142, #6302, #1719 ) ;
#6821=CARTESIAN_POINT ( 'NONE',  ( -9.421158911257350610, -6.091526235802759537, 37.92262462108629961 ) ) ;
#6822=ORIENTED_EDGE ( 'NONE', *, *, #3050, .T. ) ;
#6832=CARTESIAN_POINT ( 'NONE',  ( 9.934199572794879529, 1.970741329907451878, 41.40042185314993617 ) ) ;
#6835=CARTESIAN_POINT ( 'NONE',  ( -5.492748336992913316, -15.00000000000000000, 28.77311788903328704 ) ) ;
#6841=ADVANCED_FACE ( 'NONE', ( #3311 ), #4853, .T. ) ;
#6844=CARTESIAN_POINT ( 'NONE',  ( 0.000000000000000000, -10.00000000000000533, 0.000000000000000000 ) ) ;
#6848=CARTESIAN_POINT ( 'NONE',  ( 1.773160951616444825, -14.99999999999999822, 30.27161250924837432 ) ) ;
#6857=CARTESIAN_POINT ( 'NONE',  ( 12.09670444263329081, -2.948796042164175457, 37.07695828027222973 ) ) ;
#6859=VECTOR ( 'NONE', #6280, 1000.000000000000000 ) ;
#6884=CARTESIAN_POINT ( 'NONE',  ( 9.095951983579540823, -0.8728861028336062367, 41.83160227757072391 ) ) ;
#6889=ORIENTED_EDGE ( 'NONE', *, *, #7554, .T. ) ;
#6899=( BOUNDED_SURFACE ( )  B_SPLINE_SURFACE ( 3, 2, ( 
 ( #2281, #29, #9166 ),
 ( #5315, #8418, #8325 ),
 ( #1557, #1647, #3928 ),
 ( #867, #4573, #9119 ),
 ( #4676, #7581, #817 ),
 ( #3825, #82, #6920 ),
 ( #3074, #917, #181 ),
 ( #6092, #2426, #6182 ),
 ( #961, #9213, #5463 ),
 ( #3977, #9352, #8623 ),
 ( #1009, #5653, #9261 ),
 ( #3268, #1845, #4911 ),
 ( #8565, #5509, #322 ),
 ( #4958, #7224, #7775 ),
 ( #2571, #2474, #8664 ),
 ( #4026, #4228, #2669 ),
 ( #9456, #5696, #432 ),
 ( #4076, #8712, #5600 ),
 ( #7066, #1936, #3430 ),
 ( #9411, #1888, #1157 ),
 ( #5552, #3219, #7924 ),
 ( #6429, #7971, #4175 ),
 ( #1106, #7021, #4818 ),
 ( #7829, #6236, #1210 ),
 ( #8518, #1057, #4861 ),
 ( #1747, #282, #4769 ),
 ( #6279, #9306, #2518 ),
 ( #1793, #7121, #3323 ),
 ( #4127, #7879, #6330 ),
 ( #2628, #371, #3372 ),
 ( #7171, #6380, #6577 ),
 ( #8165, #2166, #8857 ),
 ( #6621, #9598, #8956 ),
 ( #614, #5105, #5796 ),
 ( #1396, #1301, #7320 ),
 ( #8112, #5057, #8758 ),
 ( #5883, #661, #2916 ),
 ( #1987, #2869, #2125 ),
 ( #2077, #1349, #8019 ),
 ( #9496, #7268, #4316 ),
 ( #9642, #2819, #520 ),
 ( #570, #3573, #8208 ),
 ( #5010, #4271, #4373 ),
 ( #8904, #7376, #1255 ),
 ( #9692, #4466, #6667 ),
 ( #7425, #3616, #5158 ),
 ( #4413, #3667, #5933 ),
 ( #8807, #3516, #1442 ),
 ( #474, #3470, #2777 ),
 ( #2720, #6523, #5741 ) ),
 .UNSPECIFIED., .F., .F., .F. ) 
 B_SPLINE_SURFACE_WITH_KNOTS ( ( 4, 2, 2, 2, 2, 2, 2, 2, 2, 2, 2, 2, 2, 2, 2, 2, 2, 2, 2, 2, 2, 2, 2, 2, 4 ),
 ( 3, 3 ),
 ( 0.000000000000000000, 0.002954082317436974945, 0.004431123476155462634, 0.005908164634873949890, 0.008862246952310925269, 0.01033928811102941339, 0.01181632926974789978, 0.01329337042846638617, 0.01477041158718487429, 0.01772449390462185054, 0.01920153506334033866, 0.02067857622205882678, 0.02363265853949579956, 0.02510969969821428421, 0.02658674085693277234, 0.02954082317436974858, 0.03249490549180672483, 0.03397194665052521295, 0.03544898780924370107, 0.03840307012668067732, 0.03988011128539916544, 0.04135715244411765357, 0.04431123476155462981, 0.04578827592027311100, 0.04726531707899159912 ),
 ( 0.000000000000000000, 1.000000000000000000 ),
 .UNSPECIFIED. ) 
 GEOMETRIC_REPRESENTATION_ITEM ( )  RATIONAL_B_SPLINE_SURFACE ( (
 ( 1.000000000000000000, 0.7071072458330266430, 1.000000000000000000),
 ( 1.000000000000000000, 0.7071375799977841492, 1.000000000000000000),
 ( 1.000000000000000000, 0.7087768082233868450, 1.000000000000000000),
 ( 1.000000000000000000, 0.7133511096891776981, 1.000000000000000000),
 ( 1.000000000000000000, 0.7152281558699414843, 1.000000000000000000),
 ( 1.000000000000000000, 0.7196307205451061284, 1.000000000000000000),
 ( 1.000000000000000000, 0.7221538050776922235, 1.000000000000000000),
 ( 1.000000000000000000, 0.7303875016897872774, 1.000000000000000000),
 ( 1.000000000000000000, 0.7368055093867738048, 1.000000000000000000),
 ( 1.000000000000000000, 0.7471981614082632284, 1.000000000000000000),
 ( 1.000000000000000000, 0.7508065931793335146, 1.000000000000000000),
 ( 1.000000000000000000, 0.7580362069327493124, 1.000000000000000000),
 ( 1.000000000000000000, 0.7616697343507030649, 1.000000000000000000),
 ( 1.000000000000000000, 0.7688739886174045246, 1.000000000000000000),
 ( 1.000000000000000000, 0.7724449231323486931, 1.000000000000000000),
 ( 1.000000000000000000, 0.7794306818811647108, 1.000000000000000000),
 ( 1.000000000000000000, 0.7828531719709193037, 1.000000000000000000),
 ( 1.000000000000000000, 0.7926992760373742231, 1.000000000000000000),
 ( 1.000000000000000000, 0.7985472967235329733, 1.000000000000000000),
 ( 1.000000000000000000, 0.8058679620540408761, 1.000000000000000000),
 ( 1.000000000000000000, 0.8080665605449595112, 1.000000000000000000),
 ( 1.000000000000000000, 0.8119141137016852028, 1.000000000000000000),
 ( 1.000000000000000000, 0.8135638752277519758, 1.000000000000000000),
 ( 1.000000000000000000, 0.8175016275210426064, 1.000000000000000000),
 ( 1.000000000000000000, 0.8188321819205268692, 1.000000000000000000),
 ( 1.000000000000000000, 0.8188029246654022764, 1.000000000000000000),
 ( 1.000000000000000000, 0.8184514831026776793, 1.000000000000000000),
 ( 1.000000000000000000, 0.8170668779174434793, 1.000000000000000000),
 ( 1.000000000000000000, 0.8160425189860588402, 1.000000000000000000),
 ( 1.000000000000000000, 0.8120414287524539976, 1.000000000000000000),
 ( 1.000000000000000000, 0.8081376665146275950, 1.000000000000000000),
 ( 1.000000000000000000, 0.7981628223982122350, 1.000000000000000000),
 ( 1.000000000000000000, 0.7922386866413546613, 1.000000000000000000),
 ( 1.000000000000000000, 0.7824610464937379328, 1.000000000000000000),
 ( 1.000000000000000000, 0.7790505716245198498, 1.000000000000000000),
 ( 1.000000000000000000, 0.7720072585628966477, 1.000000000000000000),
 ( 1.000000000000000000, 0.7683746194114399186, 1.000000000000000000),
 ( 1.000000000000000000, 0.7575115753154673115, 1.000000000000000000),
 ( 1.000000000000000000, 0.7502382420823103804, 1.000000000000000000),
 ( 1.000000000000000000, 0.7398999340212725206, 1.000000000000000000),
 ( 1.000000000000000000, 0.7365339334704935625, 1.000000000000000000),
 ( 1.000000000000000000, 0.7301925391221738559, 1.000000000000000000),
 ( 1.000000000000000000, 0.7272302897292030055, 1.000000000000000000),
 ( 1.000000000000000000, 0.7191033356628879769, 1.000000000000000000),
 ( 1.000000000000000000, 0.7146970297638910452, 1.000000000000000000),
 ( 1.000000000000000000, 0.7101546834031202682, 1.000000000000000000),
 ( 1.000000000000000000, 0.7089943425723855830, 1.000000000000000000),
 ( 1.000000000000000000, 0.7074683247141949627, 1.000000000000000000),
 ( 1.000000000000000000, 0.7070924731818782893, 1.000000000000000000),
 ( 1.000000000000000000, 0.7071071909622612672, 1.000000000000000000) ) ) 
 REPRESENTATION_ITEM ( '' )  SURFACE ( )  );
#6904=CARTESIAN_POINT ( 'NONE',  ( 2.581953869975504023, -6.371684584926125439, 43.83179311693056945 ) ) ;
#6908=DIRECTION ( 'NONE',  ( 0.000000000000000000, 0.000000000000000000, 1.000000000000000000 ) ) ;
#6915=CARTESIAN_POINT ( 'NONE',  ( -5.055427336041082853, -5.357477219937782031, 43.34939598124812221 ) ) ;
#6920=CARTESIAN_POINT ( 'NONE',  ( -3.252605054599032819, -6.167148258234369074, 43.73125209769538202 ) ) ;
#6921=( NAMED_UNIT ( * ) SI_UNIT ( $, .STERADIAN. ) SOLID_ANGLE_UNIT ( ) );
#6932=PLANE ( 'NONE',  #3495 ) ;
#6933=CARTESIAN_POINT ( 'NONE',  ( 4.442985217580348589, 17.45059719192358116, 38.75089293311010863 ) ) ;
#6935=ORIENTED_EDGE ( 'NONE', *, *, #6063, .T. ) ;
#6937=CARTESIAN_POINT ( 'NONE',  ( -31.00000000000001066, 27.95223080783002345, 1.991564994335481398 ) ) ;
#6947=EDGE_LOOP ( 'NONE', ( #1156, #4824, #5434, #1155, #8997, #6317 ) ) ;
#6956=ORIENTED_EDGE ( 'NONE', *, *, #6531, .T. ) ;
#6958=CARTESIAN_POINT ( 'NONE',  ( -8.976219954598299466, -1.160416084251406632, 41.89115029411580338 ) ) ;
#6961=EDGE_CURVE ( 'NONE', #4074, #996, #9601, .T. ) ;
#6969=VECTOR ( 'NONE', #5029, 1000.000000000000000 ) ;
#6971=CARTESIAN_POINT ( 'NONE',  ( 6.000000000000001776, -10.00000000000000533, -26.32489316217636954 ) ) ;
#6977=LINE ( 'NONE', #9360, #3052 ) ;
#6986=DIRECTION ( 'NONE',  ( 0.000000000000000000, 0.000000000000000000, 1.000000000000000000 ) ) ;
#6993=CIRCLE ( 'NONE', #6371, 27.00000000000000355 ) ;
#6997=DIRECTION ( 'NONE',  ( -0.000000000000000000, 1.000000000000000000, -0.000000000000000000 ) ) ;
#7006=DIRECTION ( 'NONE',  ( -0.000000000000000000, -0.000000000000000000, 1.000000000000000000 ) ) ;
#7021=CARTESIAN_POINT ( 'NONE',  ( -9.682304602691038653, 0.7514046476754797643, 37.93829281883135707 ) ) ;
#7028=CARTESIAN_POINT ( 'NONE',  ( 0.000000000000000000, 3.294852476641296768, 295.0000000000000000 ) ) ;
#7041=CARTESIAN_POINT ( 'NONE',  ( 0.000000000000000000, -10.00000000000000533, 0.000000000000000000 ) ) ;
#7044=CARTESIAN_POINT ( 'NONE',  ( 0.01843853345419280837, 13.29483547765106799, 43.99999130734108377 ) ) ;
#7054=ORIENTED_EDGE ( 'NONE', *, *, #3833, .T. ) ;
#7066=CARTESIAN_POINT ( 'NONE',  ( -11.95253140555284510, -3.346676843148376435, 37.12490603789503041 ) ) ;
#7081=EDGE_CURVE ( 'NONE', #4910, #7266, #7283, .T. ) ;
#7095=DIRECTION ( 'NONE',  ( -0.000000000000000000, 1.000000000000000000, -0.000000000000000000 ) ) ;
#7096=CARTESIAN_POINT ( 'NONE',  ( -6.000000000000005329, 30.00000000000000000, -26.32489316217636954 ) ) ;
#7097=ORIENTED_EDGE ( 'NONE', *, *, #8267, .F. ) ;
#7102=CARTESIAN_POINT ( 'NONE',  ( 2.177727725415564031, -6.478184457066049617, 38.96022561987926025 ) ) ;
#7107=CARTESIAN_POINT ( 'NONE',  ( 6.000000000000007994, 27.42469319230600533, 31.00000000000000711 ) ) ;
#7111=AXIS2_PLACEMENT_3D ( 'NONE', #3739, #6734, #9076 ) ;
#7117=EDGE_LOOP ( 'NONE', ( #9682, #5823, #180, #4480 ) ) ;
#7120=VERTEX_POINT ( 'NONE', #505 ) ;
#7121=CARTESIAN_POINT ( 'NONE',  ( -9.894639143346440235, 4.799117292280135061, 37.88549633979417308 ) ) ;
#7133=DIRECTION ( 'NONE',  ( 0.000000000000000000, 0.000000000000000000, 1.000000000000000000 ) ) ;
#7134=CARTESIAN_POINT ( 'NONE',  ( 11.07761026121386294, -5.000000000000018652, 37.39366993089406321 ) ) ;
#7136=CARTESIAN_POINT ( 'NONE',  ( -30.12488991936162108, 28.28385863652523824, 6.000000000000009770 ) ) ;
#7140=CARTESIAN_POINT ( 'NONE',  ( 7.307810609882085195, 10.12862448845246277, 42.61414511801761051 ) ) ;
#7142=CARTESIAN_POINT ( 'NONE',  ( 0.000000000000000000, 30.00000000000000000, 0.000000000000000000 ) ) ;
#7145=CARTESIAN_POINT ( 'NONE',  ( -12.92730786270479371, 6.859753899161747270, 36.79536516033844151 ) ) ;
#7159=CIRCLE ( 'NONE', #8110, 29.00000000000001776 ) ;
#7161=CARTESIAN_POINT ( 'NONE',  ( -26.32489316217636954, -15.00000000000000000, -5.999999999999995559 ) ) ;
#7166=ORIENTED_EDGE ( 'NONE', *, *, #5874, .F. ) ;
#7171=CARTESIAN_POINT ( 'NONE',  ( -12.60343472940743759, 8.172595550171486423, 36.90908749395671862 ) ) ;
#7174=VECTOR ( 'NONE', #9015, 1000.000000000000000 ) ;
#7187=CARTESIAN_POINT ( 'NONE',  ( 13.15172707401184660, 5.587632569554690676, 36.71574829764672643 ) ) ;
#7195=CARTESIAN_POINT ( 'NONE',  ( 6.127821927972693317, 11.22362876687147626, 43.03694912904850867 ) ) ;
#7196=ORIENTED_EDGE ( 'NONE', *, *, #5755, .T. ) ;
#7197=FACE_OUTER_BOUND ( 'NONE', #2852, .T. ) ;
#7199=CARTESIAN_POINT ( 'NONE',  ( -10.76024444187491191, 12.20917503714134789, 37.49526129101297300 ) ) ;
#7208=CARTESIAN_POINT ( 'NONE',  ( -4.623603109644814246, -8.639161593214105039, 39.15028058075186124 ) ) ;
#7211=ADVANCED_FACE ( 'NONE', ( #3910 ), #157, .T. ) ;
#7214=FACE_OUTER_BOUND ( 'NONE', #756, .T. ) ;
#7223=EDGE_CURVE ( 'NONE', #5938, #8381, #8299, .T. ) ;
#7224=CARTESIAN_POINT ( 'NONE',  ( -6.823606946495824666, -4.058130453688225892, 38.51596139903070082 ) ) ;
#7231=VERTEX_POINT ( 'NONE', #8447 ) ;
#7233=CARTESIAN_POINT ( 'NONE',  ( 0.000000000000000000, 19.99999999999982236, 0.000000000000000000 ) ) ;
#7234=CARTESIAN_POINT ( 'NONE',  ( 13.30507877576147280, 2.992956817324265550, 36.66028305328001125 ) ) ;
#7235=DIRECTION ( 'NONE',  ( 0.000000000000000000, -0.000000000000000000, -1.000000000000000000 ) ) ;
#7248=CARTESIAN_POINT ( 'NONE',  ( 6.840980308309120517, -7.660779396856534973, 38.68949562317958879 ) ) ;
#7250=LINE ( 'NONE', #9438, #9379 ) ;
#7253=CARTESIAN_POINT ( 'NONE',  ( -6.343556221692952413, -7.892000900020214260, 38.79899860510401055 ) ) ;
#7266=VERTEX_POINT ( 'NONE', #3100 ) ;
#7268=CARTESIAN_POINT ( 'NONE',  ( -4.686466027247337074, 12.16196211887748824, 38.79096271003776053 ) ) ;
#7271=CARTESIAN_POINT ( 'NONE',  ( -5.999999999999998224, 27.42469319230601243, 31.00000000000000711 ) ) ;
#7273=EDGE_CURVE ( 'NONE', #1089, #2358, #2398, .T. ) ;
#7280=DIRECTION ( 'NONE',  ( 0.000000000000000000, 0.000000000000000000, -1.000000000000000000 ) ) ;
#7281=CYLINDRICAL_SURFACE ( 'NONE', #3164, 10.00000000000001599 ) ;
#7283=CIRCLE ( 'NONE', #7926, 5.000000000000000888 ) ;
#7286=EDGE_CURVE ( 'NONE', #960, #6115, #5675, .T. ) ;
#7291=CARTESIAN_POINT ( 'NONE',  ( 9.983264251130078648, 3.962791862995775904, 41.37336488016977398 ) ) ;
#7299=B_SPLINE_CURVE_WITH_KNOTS ( 'NONE', 3,
 ( #2975, #8269, #2220, #9751 ),
 .UNSPECIFIED., .F., .F.,
 ( 4, 4 ),
 ( 0.000000000000000000, 0.003679109433542037191 ),
 .UNSPECIFIED. ) ;
#7305=CARTESIAN_POINT ( 'NONE',  ( -2.105232674386741554, -14.99999999999968381, 36.76945403167025006 ) ) ;
#7320=CARTESIAN_POINT ( 'NONE',  ( -7.922255980087944849, 9.405859711871766393, 42.36613572011585660 ) ) ;
#7329=CARTESIAN_POINT ( 'NONE',  ( -6.000000000000005329, -10.00000000000000533, -31.00000000000000711 ) ) ;
#7342=AXIS2_PLACEMENT_3D ( 'NONE', #5553, #4960, #2722 ) ;
#7351=CARTESIAN_POINT ( 'NONE',  ( -31.00000000000000711, 27.42469319230601243, -5.999999999999996447 ) ) ;
#7353=ADVANCED_FACE ( 'NONE', ( #9287 ), #3404, .F. ) ;
#7358=ORIENTED_EDGE ( 'NONE', *, *, #4998, .T. ) ;
#7364=DIRECTION ( 'NONE',  ( 0.000000000000000000, 0.000000000000000000, -1.000000000000000000 ) ) ;
#7367=CARTESIAN_POINT ( 'NONE',  ( 6.624374116212009334, 10.81446379339695874, 42.86925100779671993 ) ) ;
#7371=ORIENTED_EDGE ( 'NONE', *, *, #2970, .T. ) ;
#7376=CARTESIAN_POINT ( 'NONE',  ( -2.734912810787019311, 12.94483271673466440, 38.93811822664099509 ) ) ;
#7385=DIRECTION ( 'NONE',  ( -0.000000000000000000, -0.000000000000000000, 1.000000000000000000 ) ) ;
#7389=B_SPLINE_CURVE_WITH_KNOTS ( 'NONE', 3,
 ( #9130, #8429, #4688, #926, #3938, #6933, #193, #3185, #6197, #7985, #6438, #1946, #1901, #536, #6537, #1266, #8676, #484, #9560, #8030, #1221, #5664, #5806, #4237, #8725, #7187, #8077, #7934, #7234, #8772, #3384, #2583, #1315, #9363, #3483, #4872, #4922, #1168, #5615, #7134 ),
 .UNSPECIFIED., .F., .F.,
 ( 4, 2, 2, 2, 2, 2, 2, 2, 2, 2, 2, 2, 2, 2, 2, 2, 2, 2, 2, 4 ),
 ( 0.04534133810020674754, 0.04730715269063350686, 0.04927296728106025925, 0.05123878187148701857, 0.05222168916670039129, 0.05320459646191377096, 0.05517041105234051640, 0.05615331834755388912, 0.05713622564276726185, 0.06106785482362075967, 0.06205076211883412546, 0.06303366941404750512, 0.06499948400447425056, 0.06696529859490098213, 0.06893111318532772758, 0.07089692777575447302, 0.07286274236618120459, 0.07482855695660795003, 0.07581146425182133664, 0.07679437154703469548 ),
 .UNSPECIFIED. ) ;
#7398=B_SPLINE_CURVE_WITH_KNOTS ( 'NONE', 3,
 ( #2891, #8936, #2189, #1422, #7449, #8236, #1465, #4490 ),
 .UNSPECIFIED., .F., .F.,
 ( 4, 2, 2, 4 ),
 ( 8.673617379884035472E-19, 0.006005055813302546432, 0.009007583719953818346, 0.01201011162660509113 ),
 .UNSPECIFIED. ) ;
#7399=DIRECTION ( 'NONE',  ( 0.000000000000000000, -1.000000000000000000, 0.000000000000000000 ) ) ;
#7400=B_SPLINE_CURVE_WITH_KNOTS ( 'NONE', 3,
 ( #8941, #8149, #2704, #6601, #1379 ),
 .UNSPECIFIED., .F., .F.,
 ( 4, 1, 4 ),
 ( 0.04531639312264377356, 0.04532886561142526055, 0.04534133810020674754 ),
 .UNSPECIFIED. ) ;
#7404=AXIS2_PLACEMENT_3D ( 'NONE', #5259, #7433, #669 ) ;
#7408=CARTESIAN_POINT ( 'NONE',  ( 9.488413251914037616, -6.035962460277373154, 37.89468146663847392 ) ) ;
#7409=ORIENTED_EDGE ( 'NONE', *, *, #5757, .F. ) ;
#7413=FACE_OUTER_BOUND ( 'NONE', #1985, .T. ) ;
#7415=CARTESIAN_POINT ( 'NONE',  ( 12.87078970757343832, 7.181859258121229495, 36.81542066095411059 ) ) ;
#7425=CARTESIAN_POINT ( 'NONE',  ( -2.159481158939806189, 18.10398488085508362, 38.94256672920901963 ) ) ;
#7433=DIRECTION ( 'NONE',  ( -0.000000000000000000, 0.000000000000000000, 1.000000000000000000 ) ) ;
#7441=CARTESIAN_POINT ( 'NONE',  ( 9.654558508304749154, 0.6683215596213600840, 41.54876850399442390 ) ) ;
#7449=CARTESIAN_POINT ( 'NONE',  ( 31.00000000000001066, 27.95223080783002345, -1.991564994335478067 ) ) ;
#7451=ORIENTED_EDGE ( 'NONE', *, *, #9262, .F. ) ;
#7453=CARTESIAN_POINT ( 'NONE',  ( 7.745102572868511004, -15.00000000000000178, 36.88861640503655792 ) ) ;
#7464=CARTESIAN_POINT ( 'NONE',  ( 9.671751807051032657, 0.7110059823529706335, 37.94088100612616898 ) ) ;
#7466=EDGE_LOOP ( 'NONE', ( #5247, #2946, #8314, #7512 ) ) ;
#7470=ORIENTED_EDGE ( 'NONE', *, *, #4998, .F. ) ;
#7473=CARTESIAN_POINT ( 'NONE',  ( -8.114530083417154316, 9.147922986853130212, 42.28388318272966018 ) ) ;
#7484=CARTESIAN_POINT ( 'NONE',  ( 10.65363874401993982, -5.269189486186425242, 37.51926849444799217 ) ) ;
#7487=CIRCLE ( 'NONE', #6527, 27.00000000000000355 ) ;
#7489=CARTESIAN_POINT ( 'NONE',  ( 9.999999999999857891, 2.629206769140929989, 41.36423575989298485 ) ) ;
#7490=CARTESIAN_POINT ( 'NONE',  ( 0.8972019489733558117, -14.99999999999999822, 30.49724508152266367 ) ) ;
#7506=ORIENTED_EDGE ( 'NONE', *, *, #3050, .F. ) ;
#7512=ORIENTED_EDGE ( 'NONE', *, *, #3597, .F. ) ;
#7513=CARTESIAN_POINT ( 'NONE',  ( 9.932836106771395279, 1.962987939473650245, 41.40115169427811992 ) ) ;
#7521=DIRECTION ( 'NONE',  ( 0.000000000000000000, 0.000000000000000000, -1.000000000000000000 ) ) ;
#7538=SHAPE_REPRESENTATION_RELATIONSHIP ( 'NONE' , 'NONE' ,  #5213, #9748 ) ;
#7540=CARTESIAN_POINT ( 'NONE',  ( 31.00000000000000711, -15.00000000000000000, -6.000000000000006217 ) ) ;
#7547=FACE_OUTER_BOUND ( 'NONE', #2310, .T. ) ;
#7549=CARTESIAN_POINT ( 'NONE',  ( 1.427024630974435215, -14.99999999999999645, 30.38141360069620234 ) ) ;
#7553=CARTESIAN_POINT ( 'NONE',  ( -3.512770744807076184, 17.76626513302256072, 38.84267909417927456 ) ) ;
#7554=EDGE_CURVE ( 'NONE', #8960, #7666, #9006, .T. ) ;
#7559=CARTESIAN_POINT ( 'NONE',  ( 2.584928722267243906, -9.213195917623087539, 39.41233310064572493 ) ) ;
#7564=CARTESIAN_POINT ( 'NONE',  ( 13.29631672938959497, 3.758523381800037200, 36.66344176870511973 ) ) ;
#7565=EDGE_CURVE ( 'NONE', #1409, #960, #2054, .T. ) ;
#7567=CARTESIAN_POINT ( 'NONE',  ( 6.000000000000001776, -15.00000000000000000, -31.00000000000000711 ) ) ;
#7572=CARTESIAN_POINT ( 'NONE',  ( -8.654999523778794668, 8.345309360148107203, 42.04488323937489724 ) ) ;
#7578=CARTESIAN_POINT ( 'NONE',  ( -1.061959934010897166, -9.435780383690808293, 39.51211129341553630 ) ) ;
#7581=CARTESIAN_POINT ( 'NONE',  ( -2.212457605706169339, -6.470654839585223250, 38.95887210749778973 ) ) ;
#7592=CARTESIAN_POINT ( 'NONE',  ( 8.476794693501936706, -2.020196700696827108, 42.12368207434300160 ) ) ;
#7595=CARTESIAN_POINT ( 'NONE',  ( 0.000000000000000000, 3.294852476641296768, 295.0000000000000000 ) ) ;
#7600=PRODUCT_DEFINITION_FORMATION_WITH_SPECIFIED_SOURCE ( 'ANY', '', #8602, .NOT_KNOWN. ) ;
#7605=CARTESIAN_POINT ( 'NONE',  ( 2.461798344461688437, -15.00000000000000000, 30.03527913442230712 ) ) ;
#7606=VERTEX_POINT ( 'NONE', #6971 ) ;
#7611=CARTESIAN_POINT ( 'NONE',  ( 9.331651614526968785, -0.3404697570833234432, 38.02245871504709385 ) ) ;
#7617=CARTESIAN_POINT ( 'NONE',  ( 0.000000000000000000, 3.294852476641296768, 184.6745183374407020 ) ) ;
#7619=CARTESIAN_POINT ( 'NONE',  ( 6.000000000000001776, 30.00000000000000000, -28.37252191822216218 ) ) ;
#7628=CARTESIAN_POINT ( 'NONE',  ( -0.02945139436736224012, -11.70511861050984947, 43.99999014335539016 ) ) ;
#7643=CARTESIAN_POINT ( 'NONE',  ( -31.00000000000000711, -15.00000000000000000, 6.000000000000009770 ) ) ;
#7651=CARTESIAN_POINT ( 'NONE',  ( 26.32489316217636954, -10.00000000000000533, -6.000000000000006217 ) ) ;
#7653=VERTEX_POINT ( 'NONE', #2334 ) ;
#7662=CARTESIAN_POINT ( 'NONE',  ( 6.656046503713715090, -9.726635889951044334, 38.43478818343638181 ) ) ;
#7666=VERTEX_POINT ( 'NONE', #3123 ) ;
#7676=CARTESIAN_POINT ( 'NONE',  ( -9.656652801210938719, 0.6761216413562457506, 41.54767058179530181 ) ) ;
#7688=ORIENTED_EDGE ( 'NONE', *, *, #93, .T. ) ;
#7711=CARTESIAN_POINT ( 'NONE',  ( 2.263813592557596177, -6.451033302730273533, 43.87142663822828581 ) ) ;
#7714=CARTESIAN_POINT ( 'NONE',  ( 5.008074634385683233, 27.61318074145109591, 31.00000000000000355 ) ) ;
#7718=ORIENTED_EDGE ( 'NONE', *, *, #5710, .T. ) ;
#7725=DIRECTION ( 'NONE',  ( 0.9999978484633867959, -0.001963425851322921859, 0.0006693485817986371015 ) ) ;
#7729=ORIENTED_EDGE ( 'NONE', *, *, #9331, .F. ) ;
#7755=EDGE_CURVE ( 'NONE', #4074, #8381, #434, .T. ) ;
#7758=VERTEX_POINT ( 'NONE', #324 ) ;
#7766=DIRECTION ( 'NONE',  ( 0.000000000000000000, 0.000000000000000000, 1.000000000000000000 ) ) ;
#7773=ORIENTED_EDGE ( 'NONE', *, *, #4986, .T. ) ;
#7775=CARTESIAN_POINT ( 'NONE',  ( -7.316365616915794234, -3.529765552624353209, 42.61083985122122897 ) ) ;
#7776=VECTOR ( 'NONE', #8644, 1000.000000000000000 ) ;
#7777=AXIS2_PLACEMENT_3D ( 'NONE', #6405, #3948, #2453 ) ;
#7793=CARTESIAN_POINT ( 'NONE',  ( -8.237197373723139648, -15.00000000000000000, 27.80554943579302929 ) ) ;
#7800=VECTOR ( 'NONE', #9082, 1000.000000000000000 ) ;
#7808=CARTESIAN_POINT ( 'NONE',  ( -31.00000000000000711, -10.00000000000000533, -5.999999999999996447 ) ) ;
#7817=MECHANICAL_DESIGN_GEOMETRIC_PRESENTATION_REPRESENTATION('',(#6071),#6235);
#7818=EDGE_CURVE ( 'NONE', #5073, #9521, #9121, .T. ) ;
#7819=CARTESIAN_POINT ( 'NONE',  ( 31.00000000000000711, -15.00000000000000000, -6.000000000000006217 ) ) ;
#7828=CIRCLE ( 'NONE', #1041, 39.00000000000002132 ) ;
#7829=CARTESIAN_POINT ( 'NONE',  ( -13.21233427609164934, 1.350469624994050211, 36.69423386285060928 ) ) ;
#7845=DIRECTION ( 'NONE',  ( 0.000000000000000000, -1.000000000000000000, 0.000000000000000000 ) ) ;
#7849=B_SPLINE_CURVE_WITH_KNOTS ( 'NONE', 3,
 ( #3545, #4150, #9577, #2795, #9376, #5816, #2600, #8831, #4843, #4101, #1865, #7145, #1914, #4937, #7949, #7998, #7199, #1179, #4201, #735, #9722, #2944, #5905, #7553, #9029, #6738, #6687, #2889, #5224, #2098 ),
 .UNSPECIFIED., .F., .F.,
 ( 4, 2, 2, 2, 2, 2, 2, 2, 2, 2, 2, 2, 2, 2, 4 ),
 ( 0.01382556044152182841, 0.01776191452666206830, 0.01973009156923219085, 0.02169826861180230992, 0.02366644565437243247, 0.02563462269694255502, 0.02760279973951267757, 0.02957097678208280012, 0.03350733086722303827, 0.03744368495236328337, 0.03941186199493340592, 0.04138003903750352847, 0.04236412755878859321, 0.04334821608007365101, 0.04531639312264377356 ),
 .UNSPECIFIED. ) ;
#7862=CARTESIAN_POINT ( 'NONE',  ( 2.735220335096864019, -6.341052613831273277, 38.93530391522555334 ) ) ;
#7867=CARTESIAN_POINT ( 'NONE',  ( 4.007938479032607582, 27.75794689997811204, 31.00000000000000000 ) ) ;
#7869=CARTESIAN_POINT ( 'NONE',  ( 0.000000000000000000, 3.294852476641296768, 300.0000000000000000 ) ) ;
#7879=CARTESIAN_POINT ( 'NONE',  ( -9.832659897753353917, 5.164632082215160125, 37.90110321522534065 ) ) ;
#7892=CARTESIAN_POINT ( 'NONE',  ( -31.00000000000000711, 27.42469319230600533, 6.000000000000009770 ) ) ;
#7894=AXIS2_PLACEMENT_3D ( 'NONE', #2088, #6586, #6437 ) ;
#7901=ORIENTED_EDGE ( 'NONE', *, *, #4508, .T. ) ;
#7912=ORIENTED_EDGE ( 'NONE', *, *, #5522, .T. ) ;
#7919=EDGE_LOOP ( 'NONE', ( #8238, #4559, #5981, #4647, #6265 ) ) ;
#7924=CARTESIAN_POINT ( 'NONE',  ( -9.473662127245630060, 0.07647080102255582323, 41.64234459406086586 ) ) ;
#7926=AXIS2_PLACEMENT_3D ( 'NONE', #1973, #2156, #1243 ) ;
#7928=VERTEX_POINT ( 'NONE', #6669 ) ;
#7934=CARTESIAN_POINT ( 'NONE',  ( 13.30448870009049323, 3.640525045295374795, 36.66049983383106792 ) ) ;
#7945=CARTESIAN_POINT ( 'NONE',  ( 8.649757686324669237, 8.323462134889155095, 42.04423075653439668 ) ) ;
#7947=CARTESIAN_POINT ( 'NONE',  ( 0.000000000000000000, 3.294852476641296768, 300.0000000000000000 ) ) ;
#7949=CARTESIAN_POINT ( 'NONE',  ( -12.18343812368627255, 9.336105043037195017, 37.04911908969401679 ) ) ;
#7950=CARTESIAN_POINT ( 'NONE',  ( 5.468730748236366068, -8.297078842874196170, 38.99054534826768048 ) ) ;
#7957=CARTESIAN_POINT ( 'NONE',  ( -3.817146860096892524, -15.00000000000000000, 29.48174236496974032 ) ) ;
#7962=CARTESIAN_POINT ( 'NONE',  ( 6.823105196324329214, 10.64845247602661082, 38.51605970865411877 ) ) ;
#7971=CARTESIAN_POINT ( 'NONE',  ( -9.581830020199642917, 0.3921576626816477562, 37.96287317033787900 ) ) ;
#7976=CARTESIAN_POINT ( 'NONE',  ( -5.999999999999998224, 29.14236109046821710, 29.24912810952613640 ) ) ;
#7981=AXIS2_PLACEMENT_3D ( 'NONE', #8067, #9745, #4374 ) ;
#7983=CARTESIAN_POINT ( 'NONE',  ( 0.000000000000000000, -15.00000000000000000, -29.00000000000001776 ) ) ;
#7985=CARTESIAN_POINT ( 'NONE',  ( 6.715732449718500696, 16.24544142831953053, 38.41843156493658995 ) ) ;
#7998=CARTESIAN_POINT ( 'NONE',  ( -11.40964930878180539, 11.10725308166288983, 37.29763346372921262 ) ) ;
#7999=ADVANCED_FACE ( 'NONE', ( #3618 ), #2877, .T. ) ;
#8005=CARTESIAN_POINT ( 'NONE',  ( -0.3713926049973746979, -15.00000000000000000, 30.56995792405530921 ) ) ;
#8012=CARTESIAN_POINT ( 'NONE',  ( 8.498720194445880338, 8.574681387762774776, 42.11372032734551141 ) ) ;
#8019=CARTESIAN_POINT ( 'NONE',  ( -6.094378065318124982, 11.24985937468323272, 43.04782701210960028 ) ) ;
#8020=DIRECTION ( 'NONE',  ( -0.000000000000000000, 1.000000000000000000, -0.000000000000000000 ) ) ;
#8022=ORIENTED_EDGE ( 'NONE', *, *, #2983, .F. ) ;
#8024=CARTESIAN_POINT ( 'NONE',  ( 0.000000000000000000, 30.00000000000000000, 0.000000000000000000 ) ) ;
#8025=ORIENTED_EDGE ( 'NONE', *, *, #2970, .F. ) ;
#8028=LINE ( 'NONE', #2086, #5742 ) ;
#8030=CARTESIAN_POINT ( 'NONE',  ( 12.05879450961799293, 9.620832044272598083, 37.08913302436281612 ) ) ;
#8047=CARTESIAN_POINT ( 'NONE',  ( -6.507333377502796168, -14.99999999999967848, 36.82578466839068909 ) ) ;
#8053=CARTESIAN_POINT ( 'NONE',  ( 5.532933570186216343, 16.94308342398178269, 38.60764366510559853 ) ) ;
#8055=EDGE_CURVE ( 'NONE', #8381, #7653, #55, .T. ) ;
#8067=CARTESIAN_POINT ( 'NONE',  ( 0.000000000000000000, 3.294852476641296768, 294.6136752714472777 ) ) ;
#8070=EDGE_CURVE ( 'NONE', #1345, #1203, #9207, .T. ) ;
#8077=CARTESIAN_POINT ( 'NONE',  ( 13.22768554207220681, 4.942043779154436933, 36.68828154652676687 ) ) ;
#8085=CARTESIAN_POINT ( 'NONE',  ( 8.483224498846656303, 8.599388824895884298, 42.12074175542014132 ) ) ;
#8089=FACE_OUTER_BOUND ( 'NONE', #6482, .T. ) ;
#8090=VECTOR ( 'NONE', #6818, 1000.000000000000000 ) ;
#8097=CARTESIAN_POINT ( 'NONE',  ( -7.237833666954393230, -7.422220416173621160, 38.57360862901651188 ) ) ;
#8100=DIRECTION ( 'NONE',  ( 1.000000000000000000, 0.000000000000000000, 0.000000000000000000 ) ) ;
#8102=CARTESIAN_POINT ( 'NONE',  ( 7.068415056849144840, 10.41224345616790892, 38.47601730954646371 ) ) ;
#8110=AXIS2_PLACEMENT_3D ( 'NONE', #2243, #1424, #9088 ) ;
#8112=CARTESIAN_POINT ( 'NONE',  ( -9.980720655645276551, 13.21681672747774883, 37.70234918754850639 ) ) ;
#8114=EDGE_CURVE ( 'NONE', #2298, #1381, #3817, .T. ) ;
#8116=AXIS2_PLACEMENT_3D ( 'NONE', #9619, #2842, #8880 ) ;
#8125=FACE_OUTER_BOUND ( 'NONE', #2907, .T. ) ;
#8147=PRODUCT_DEFINITION ( 'UNKNOWN', '', #7600, #2771 ) ;
#8149=CARTESIAN_POINT ( 'NONE',  ( 0.004085762815451446546, 18.29485247664131009, 39.00000000000001421 ) ) ;
#8150=CARTESIAN_POINT ( 'NONE',  ( -9.224918227939335580, -6.208428183824680424, 37.97970803284726315 ) ) ;
#8154=DIRECTION ( 'NONE',  ( -1.000000000000000000, 0.000000000000000000, 0.000000000000000000 ) ) ;
#8155=ORIENTED_EDGE ( 'NONE', *, *, #9513, .T. ) ;
#8156=CARTESIAN_POINT ( 'NONE',  ( 7.535708689751818845, 9.876535171860036044, 42.52448306728676641 ) ) ;
#8165=CARTESIAN_POINT ( 'NONE',  ( -11.92603897288437054, 9.998747279519278663, 37.13350106079722934 ) ) ;
#8168=EDGE_LOOP ( 'NONE', ( #6180, #5713, #5671, #5447 ) ) ;
#8175=B_SPLINE_CURVE_WITH_KNOTS ( 'NONE', 3,
 ( #6364, #8600, #1831, #7867, #7714, #7107 ),
 .UNSPECIFIED., .F., .F.,
 ( 4, 2, 4 ),
 ( 0.006018989108141226639, 0.009014550367373157583, 0.01201011162660509113 ),
 .UNSPECIFIED. ) ;
#8183=DIRECTION ( 'NONE',  ( -1.000000000000000000, 0.000000000000000000, 0.000000000000000000 ) ) ;
#8188=DIRECTION ( 'NONE',  ( 0.000000000000000000, 0.000000000000000000, -1.000000000000000000 ) ) ;
#8189=AXIS2_PLACEMENT_3D ( 'NONE', #7233, #8675, #7280 ) ;
#8193=CARTESIAN_POINT ( 'NONE',  ( 9.147656056445134354, -14.99999999999968558, 37.02405928711753802 ) ) ;
#8199=CARTESIAN_POINT ( 'NONE',  ( 7.509679877969126949, -3.381201913332376741, 38.40166088718918047 ) ) ;
#8201=CARTESIAN_POINT ( 'NONE',  ( -11.07761026121387538, -4.999999999999996447, 37.39366993089406321 ) ) ;
#8208=CARTESIAN_POINT ( 'NONE',  ( -4.420886993428805312, 12.27057209469446875, 43.49964545912311564 ) ) ;
#8210=DIRECTION ( 'NONE',  ( 1.000000000000000000, 0.000000000000000000, 0.000000000000000000 ) ) ;
#8219=DIRECTION ( 'NONE',  ( 1.000000000000000000, 0.000000000000000000, 0.000000000000000000 ) ) ;
#8226=CARTESIAN_POINT ( 'NONE',  ( 9.737280834746197655, 0.9936006834773455365, 41.50515603427665923 ) ) ;
#8236=CARTESIAN_POINT ( 'NONE',  ( 31.00000000000001066, 27.75862132583096553, -4.003261267919809185 ) ) ;
#8238=ORIENTED_EDGE ( 'NONE', *, *, #916, .F. ) ;
#8242=CIRCLE ( 'NONE', #6819, 27.00000000000000355 ) ;
#8246=DIRECTION ( 'NONE',  ( 1.000000000000000000, 0.000000000000000000, 0.000000000000000000 ) ) ;
#8247=ORIENTED_EDGE ( 'NONE', *, *, #8799, .F. ) ;
#8250=CARTESIAN_POINT ( 'NONE',  ( 13.18962522851849251, 5.248138163192250794, 36.70198719095098028 ) ) ;
#8266=VERTEX_POINT ( 'NONE', #1836 ) ;
#8267=EDGE_CURVE ( 'NONE', #4918, #1718, #3313, .T. ) ;
#8269=CARTESIAN_POINT ( 'NONE',  ( 6.000000000000001776, 29.14236109046821710, -29.24912810952613640 ) ) ;
#8272=AXIS2_PLACEMENT_3D ( 'NONE', #5955, #8934, #1520 ) ;
#8279=CARTESIAN_POINT ( 'NONE',  ( 8.646527988035350276, -1.739381284455594923, 42.04573165431521176 ) ) ;
#8281=CARTESIAN_POINT ( 'NONE',  ( -0.7306063396721927949, -15.00000000000000000, 30.53418880813659086 ) ) ;
#8283=ORIENTED_EDGE ( 'NONE', *, *, #9140, .T. ) ;
#8284=CARTESIAN_POINT ( 'NONE',  ( 6.000000000000007994, -10.00000000000000533, 26.32489316217636954 ) ) ;
#8285=VECTOR ( 'NONE', #1689, 1000.000000000000000 ) ;
#8291=PLANE ( 'NONE',  #3375 ) ;
#8297=CARTESIAN_POINT ( 'NONE',  ( 1.945897168356747864, -15.00000000000000000, 30.21518419675670586 ) ) ;
#8299=LINE ( 'NONE', #2250, #8722 ) ;
#8303=CARTESIAN_POINT ( 'NONE',  ( 13.29364790190014212, 2.276109693707590420, 36.66440956898404124 ) ) ;
#8306=DIRECTION ( 'NONE',  ( -0.000000000000000000, 1.000000000000000000, -0.000000000000000000 ) ) ;
#8309=DIRECTION ( 'NONE',  ( 0.000000000000000000, 0.000000000000000000, -1.000000000000000000 ) ) ;
#8313=EDGE_CURVE ( 'NONE', #1203, #5506, #6227, .T. ) ;
#8314=ORIENTED_EDGE ( 'NONE', *, *, #9744, .T. ) ;
#8315=CARTESIAN_POINT ( 'NONE',  ( -9.999999999999436895, 3.627100512255909681, 41.36423575989321222 ) ) ;
#8325=CARTESIAN_POINT ( 'NONE',  ( -0.6856205131675365827, -6.703820630692375993, 43.99932147620603473 ) ) ;
#8328=ORIENTED_EDGE ( 'NONE', *, *, #8070, .F. ) ;
#8334=DIRECTION ( 'NONE',  ( -1.000000000000000000, 0.000000000000000000, 0.000000000000000000 ) ) ;
#8339=B_SPLINE_CURVE_WITH_KNOTS ( 'NONE', 3,
 ( #805, #4560, #1596, #3012, #9152, #4053 ),
 .UNSPECIFIED., .F., .F.,
 ( 4, 2, 4 ),
 ( 0.006018989108141225772, 0.009014550367373161052, 0.01201011162660509460 ),
 .UNSPECIFIED. ) ;
#8340=DIRECTION ( 'NONE',  ( -0.000000000000000000, 0.000000000000000000, 1.000000000000000000 ) ) ;
#8343=CARTESIAN_POINT ( 'NONE',  ( 3.810735843230694364, -15.00000000000000000, 29.48446022066782035 ) ) ;
#8347=DIRECTION ( 'NONE',  ( -0.000000000000000000, -0.000000000000000000, 1.000000000000000000 ) ) ;
#8349=CARTESIAN_POINT ( 'NONE',  ( 12.94589496447643739, -0.1577490691376046139, 36.78875203023495999 ) ) ;
#8351=ORIENTED_EDGE ( 'NONE', *, *, #3833, .F. ) ;
#8352=DIRECTION ( 'NONE',  ( -0.000000000000000000, 1.000000000000000000, -0.000000000000000000 ) ) ;
#8353=LINE ( 'NONE', #1688, #6137 ) ;
#8358=CARTESIAN_POINT ( 'NONE',  ( -8.964960879312730668, 7.774309358726588570, 41.89665171198695504 ) ) ;
#8359=AXIS2_PLACEMENT_3D ( 'NONE', #6844, #2489, #3092 ) ;
#8368=CARTESIAN_POINT ( 'NONE',  ( -0.5436840601780645876, -9.469167920862840759, 39.52694059679008376 ) ) ;
#8372=DIRECTION ( 'NONE',  ( 0.000000000000000000, 0.000000000000000000, -1.000000000000000000 ) ) ;
#8381=VERTEX_POINT ( 'NONE', #2900 ) ;
#8382=CARTESIAN_POINT ( 'NONE',  ( 3.237977208914636140, -6.172201048711161597, 43.73371347798987330 ) ) ;
#8384=DIRECTION ( 'NONE',  ( 0.000000000000000000, 0.000000000000000000, -1.000000000000000000 ) ) ;
#8388=CIRCLE ( 'NONE', #5545, 39.00000000000002132 ) ;
#8394=CARTESIAN_POINT ( 'NONE',  ( 5.490675478207040605, -15.00000000000000000, 28.78002780014356077 ) ) ;
#8395=EDGE_CURVE ( 'NONE', #1760, #2374, #8762, .T. ) ;
#8400=ORIENTED_EDGE ( 'NONE', *, *, #3630, .T. ) ;
#8401=CARTESIAN_POINT ( 'NONE',  ( 10.00064848029234632, 3.603966413413724368, 41.36388302110313475 ) ) ;
#8405=LINE ( 'NONE', #800, #8285 ) ;
#8412=AXIS2_PLACEMENT_3D ( 'NONE', #2748, #3637, #5672 ) ;
#8417=EDGE_LOOP ( 'NONE', ( #136, #1887, #8560, #4497, #2389 ) ) ;
#8418=CARTESIAN_POINT ( 'NONE',  ( -0.5685535372354538763, -6.704273290862945878, 38.99985098249960913 ) ) ;
#8422=ORIENTED_EDGE ( 'NONE', *, *, #3312, .F. ) ;
#8425=CARTESIAN_POINT ( 'NONE',  ( 2.284773941623177151, -6.446222133925260778, 43.86901922224630823 ) ) ;
#8427=EDGE_CURVE ( 'NONE', #9075, #1923, #2157, .T. ) ;
#8429=CARTESIAN_POINT ( 'NONE',  ( 0.6684956564278037305, 18.29348733819152528, 38.99958749751832698 ) ) ;
#8433=ORIENTED_EDGE ( 'NONE', *, *, #916, .T. ) ;
#8442=CARTESIAN_POINT ( 'NONE',  ( 31.00000000000000711, -10.00000000000000533, 6.000000000000000000 ) ) ;
#8447=CARTESIAN_POINT ( 'NONE',  ( 6.000000000000007994, 27.42469319230600533, 31.00000000000000711 ) ) ;
#8453=CARTESIAN_POINT ( 'NONE',  ( 4.270857271783432552, -10.91876588853619445, 38.76773248714805931 ) ) ;
#8465=CARTESIAN_POINT ( 'NONE',  ( 26.32489316217636954, 30.00000000000000000, -6.000000000000006217 ) ) ;
#8470=ORIENTED_EDGE ( 'NONE', *, *, #6475, .F. ) ;
#8477=VERTEX_POINT ( 'NONE', #8843 ) ;
#8485=CARTESIAN_POINT ( 'NONE',  ( -31.00000000000000711, -10.00000000000000533, 6.000000000000009770 ) ) ;
#8488=ADVANCED_FACE ( 'NONE', ( #7413 ), #3504, .T. ) ;
#8489=EDGE_CURVE ( 'NONE', #7928, #6799, #519, .T. ) ;
#8494=ORIENTED_EDGE ( 'NONE', *, *, #2997, .F. ) ;
#8509=CARTESIAN_POINT ( 'NONE',  ( -5.861437416230651287, -4.813697954704956317, 43.11457445622953344 ) ) ;
#8518=CARTESIAN_POINT ( 'NONE',  ( -13.29668680294569683, 2.328753113016122533, 36.66330756792502399 ) ) ;
#8524=ORIENTED_EDGE ( 'NONE', *, *, #7223, .F. ) ;
#8531=ADVANCED_FACE ( 'NONE', ( #9142 ), #576, .T. ) ;
#8532=EDGE_CURVE ( 'NONE', #577, #9341, #4834, .T. ) ;
#8533=CYLINDRICAL_SURFACE ( 'NONE', #4962, 27.00000000000000355 ) ;
#8540=B_SPLINE_CURVE_WITH_KNOTS ( 'NONE', 3,
 ( #7892, #7136, #3387, #539 ),
 .UNSPECIFIED., .F., .F.,
 ( 4, 4 ),
 ( 9.813077866773594792E-18, 0.003679109433542027217 ),
 .UNSPECIFIED. ) ;
#8545=CARTESIAN_POINT ( 'NONE',  ( 3.852137862560303105, -5.973899105776613538, 38.86704162447477273 ) ) ;
#8560=ORIENTED_EDGE ( 'NONE', *, *, #1418, .F. ) ;
#8565=CARTESIAN_POINT ( 'NONE',  ( -9.120756353288166807, -7.629869846859943294, 37.91977750705790129 ) ) ;
#8577=DIRECTION ( 'NONE',  ( -1.000000000000000000, 0.000000000000000000, 0.000000000000000000 ) ) ;
#8579=CARTESIAN_POINT ( 'NONE',  ( 6.000000000000001776, -10.00000000000000533, -31.00000000000000711 ) ) ;
#8582=CARTESIAN_POINT ( 'NONE',  ( 0.000000000000000000, -15.00000000000000000, 0.000000000000000000 ) ) ;
#8587=CARTESIAN_POINT ( 'NONE',  ( -3.246812748820610661, 12.77555213868837569, 43.73912123486446291 ) ) ;
#8592=CARTESIAN_POINT ( 'NONE',  ( 6.000000000000007994, -10.00000000000000533, 31.00000000000000711 ) ) ;
#8593=CARTESIAN_POINT ( 'NONE',  ( 5.225835130983021770, -5.267432217960810625, 38.73366001166045436 ) ) ;
#8594=CARTESIAN_POINT ( 'NONE',  ( -28.37252191822215863, 30.00000000000000000, 6.000000000000009770 ) ) ;
#8596=CIRCLE ( 'NONE', #9385, 28.99999999999995026 ) ;
#8597=VERTEX_POINT ( 'NONE', #3753 ) ;
#8600=CARTESIAN_POINT ( 'NONE',  ( 0.9994180975881575835, 27.99999999999992184, 31.00000000000001066 ) ) ;
#8602=PRODUCT ( 'Lever with a Die for Securing the Metal Body', 'Lever with a Die for Securing the Metal Body', '', ( #4504 ) ) ;
#8608=AXIS2_PLACEMENT_3D ( 'NONE', #4574, #3075, #182 ) ;
#8609=EDGE_CURVE ( 'NONE', #1828, #4609, #1084, .T. ) ;
#8623=CARTESIAN_POINT ( 'NONE',  ( -5.854220575332682586, -4.818998781743923487, 43.11681015548058582 ) ) ;
#8631=CARTESIAN_POINT ( 'NONE',  ( 26.32489316217636954, -10.00000000000000533, -6.000000000000006217 ) ) ;
#8632=CARTESIAN_POINT ( 'NONE',  ( -6.000000000000005329, -15.00000000000000000, -26.32489316217636954 ) ) ;
#8633=CARTESIAN_POINT ( 'NONE',  ( 0.000000000000000000, 30.00000000000000000, 0.000000000000000000 ) ) ;
#8637=ORIENTED_EDGE ( 'NONE', *, *, #2983, .T. ) ;
#8644=DIRECTION ( 'NONE',  ( 1.000000000000000000, 0.000000000000000000, 0.000000000000000000 ) ) ;
#8646=CARTESIAN_POINT ( 'NONE',  ( 6.587360613405085275, -4.236025479845884512, 42.87792995678174890 ) ) ;
#8652=APPLICATION_CONTEXT ( 'automotive_design' ) ;
#8664=CARTESIAN_POINT ( 'NONE',  ( -7.533180272099675001, -3.289707944753238245, 42.52548976219601684 ) ) ;
#8669=AXIS2_PLACEMENT_3D ( 'NONE', #1167, #442, #9467 ) ;
#8675=DIRECTION ( 'NONE',  ( -0.000000000000000000, -1.000000000000000000, -0.000000000000000000 ) ) ;
#8676=CARTESIAN_POINT ( 'NONE',  ( 9.780907758090382487, 13.46073421343169052, 37.75414574899522790 ) ) ;
#8692=DIRECTION ( 'NONE',  ( 0.000000000000000000, 0.000000000000000000, -1.000000000000000000 ) ) ;
#8700=CARTESIAN_POINT ( 'NONE',  ( -5.552440503301123265, -15.00000000000030909, 36.79988656443232742 ) ) ;
#8704=CARTESIAN_POINT ( 'NONE',  ( 1.109999172770812503, 13.23925573637847997, 38.99045641393601613 ) ) ;
#8706=VECTOR ( 'NONE', #3788, 1000.000000000000000 ) ;
#8712=CARTESIAN_POINT ( 'NONE',  ( -8.387767640013615633, -2.225892194537749447, 38.23251940671359250 ) ) ;
#8720=EDGE_LOOP ( 'NONE', ( #456, #6329, #1078, #9309 ) ) ;
#8722=VECTOR ( 'NONE', #5436, 1000.000000000000000 ) ;
#8725=CARTESIAN_POINT ( 'NONE',  ( 12.92792341719169791, 6.856606603030884983, 36.79514769918270645 ) ) ;
#8737=DIRECTION ( 'NONE',  ( -0.000000000000000000, -0.000000000000000000, 1.000000000000000000 ) ) ;
#8742=ORIENTED_EDGE ( 'NONE', *, *, #4508, .F. ) ;
#8745=ORIENTED_EDGE ( 'NONE', *, *, #2997, .T. ) ;
#8749=CARTESIAN_POINT ( 'NONE',  ( 9.726904566720470768, 13.53265914481252885, 37.76886403029045169 ) ) ;
#8756=VERTEX_POINT ( 'NONE', #1661 ) ;
#8758=CARTESIAN_POINT ( 'NONE',  ( -7.506866817950279547, 9.909495310584443217, 42.53598369858231365 ) ) ;
#8762=CIRCLE ( 'NONE', #6067, 10.00000000000000000 ) ;
#8763=VECTOR ( 'NONE', #6581, 1000.000000000000000 ) ;
#8769=ORIENTED_EDGE ( 'NONE', *, *, #1792, .T. ) ;
#8771=FACE_OUTER_BOUND ( 'NONE', #6947, .T. ) ;
#8772=CARTESIAN_POINT ( 'NONE',  ( 13.23285520384964009, 1.704015861027379009, 36.68641462353301108 ) ) ;
#8774=B_SPLINE_CURVE_WITH_KNOTS ( 'NONE', 3,
 ( #1448, #6479, #6821, #9750, #9060, #913, #6725, #3925, #9210, #3821, #4713, #7578, #8368, #4568 ),
 .UNSPECIFIED., .F., .F.,
 ( 4, 2, 2, 2, 2, 2, 4 ),
 ( 0.000000000000000000, 0.003068295728000690944, 0.006136591456001381888, 0.007670739320001727576, 0.009204887184002075867, 0.01073903504800242069, 0.01227318291200276898 ),
 .UNSPECIFIED. ) ;
#8782=CARTESIAN_POINT ( 'NONE',  ( 8.125263811375475598, 9.132942212448577735, 42.27923313267293537 ) ) ;
#8783=EDGE_LOOP ( 'NONE', ( #8524, #8400, #6099, #658 ) ) ;
#8799=EDGE_CURVE ( 'NONE', #1409, #9349, #6618, .T. ) ;
#8800=CARTESIAN_POINT ( 'NONE',  ( 4.444319822552836641, 12.28422794470395374, 38.81412028401931025 ) ) ;
#8806=ORIENTED_EDGE ( 'NONE', *, *, #5874, .T. ) ;
#8807=CARTESIAN_POINT ( 'NONE',  ( -0.8485526577698208062, 18.27243448981633023, 38.99321009875914967 ) ) ;
#8817=LINE ( 'NONE', #443, #8846 ) ;
#8824=CARTESIAN_POINT ( 'NONE',  ( 6.000000000000007994, -15.00000000000000000, 31.00000000000000711 ) ) ;
#8825=CARTESIAN_POINT ( 'NONE',  ( 8.957468044428361864, 7.752316930812642504, 41.89900961843087401 ) ) ;
#8831=CARTESIAN_POINT ( 'NONE',  ( -13.30503757985684565, 2.990201221717010860, 36.66029814382953589 ) ) ;
#8834=DIRECTION ( 'NONE',  ( -0.000000000000000000, 1.000000000000000000, -0.000000000000000000 ) ) ;
#8837=DIRECTION ( 'NONE',  ( -0.000000000000000000, 1.000000000000000000, -0.000000000000000000 ) ) ;
#8843=CARTESIAN_POINT ( 'NONE',  ( -26.32489316217636954, -10.00000000000000533, 6.000000000000009770 ) ) ;
#8846=VECTOR ( 'NONE', #4970, 1000.000000000000000 ) ;
#8857=CARTESIAN_POINT ( 'NONE',  ( -8.970012219034815715, 7.764115678634449402, 41.89420632471620110 ) ) ;
#8861=DIRECTION ( 'NONE',  ( 0.000000000000000000, -1.000000000000000000, 0.000000000000000000 ) ) ;
#8870=LINE ( 'NONE', #7540, #7174 ) ;
#8877=CARTESIAN_POINT ( 'NONE',  ( 3.274489253962265867, 12.76606442083950910, 43.73447258638396562 ) ) ;
#8878=DIRECTION ( 'NONE',  ( 0.000000000000000000, -0.7071067811865512365, -0.7071067811865439090 ) ) ;
#8880=DIRECTION ( 'NONE',  ( 0.000000000000000000, 0.000000000000000000, -1.000000000000000000 ) ) ;
#8888=CARTESIAN_POINT ( 'NONE',  ( -0.9067368948456047129, -14.99999999999999822, 30.49541815531657818 ) ) ;
#8892=DIRECTION ( 'NONE',  ( 0.9588120495101036811, 9.854661834794498374E-17, 0.2840412887490736393 ) ) ;
#8894=CARTESIAN_POINT ( 'NONE',  ( 5.316540241612734974, 11.77069107846751095, 43.27322217794340986 ) ) ;
#8896=ORIENTED_EDGE ( 'NONE', *, *, #1288, .F. ) ;
#8900=EDGE_LOOP ( 'NONE', ( #8494, #6170, #1870, #466 ) ) ;
#8904=CARTESIAN_POINT ( 'NONE',  ( -4.284152118168920609, 17.52839865830862820, 38.77238817881250554 ) ) ;
#8911=AXIS2_PLACEMENT_3D ( 'NONE', #4208, #8834, #4992 ) ;
#8914=CARTESIAN_POINT ( 'NONE',  ( -6.000000000000005329, -10.00000000000000533, -26.32489316217636954 ) ) ;
#8931=CARTESIAN_POINT ( 'NONE',  ( -1.783505000977663846, -14.99999999999999822, 30.27207879089416664 ) ) ;
#8934=DIRECTION ( 'NONE',  ( 0.000000000000000000, -1.000000000000000000, 0.000000000000000000 ) ) ;
#8936=CARTESIAN_POINT ( 'NONE',  ( 31.00000000000000711, 27.80235549540589801, 4.012532818320192263 ) ) ;
#8941=CARTESIAN_POINT ( 'NONE',  ( 6.439978105601112524E-15, 18.29485247664131009, 39.00000000000002132 ) ) ;
#8942=CARTESIAN_POINT ( 'NONE',  ( 8.639162863793341529, -6.583298275952675915, 38.16418810910280968 ) ) ;
#8948=CARTESIAN_POINT ( 'NONE',  ( 8.149741407064750476, -2.543282342078551306, 38.27864742387711772 ) ) ;
#8956=CARTESIAN_POINT ( 'NONE',  ( -8.659653037499971617, 8.337804354671460416, 42.04276546470546805 ) ) ;
#8960=VERTEX_POINT ( 'NONE', #2365 ) ;
#8964=EDGE_CURVE ( 'NONE', #9341, #577, #9097, .T. ) ;
#8973=CARTESIAN_POINT ( 'NONE',  ( 5.030598735306972102, -5.371835421513210029, 43.35589067224919546 ) ) ;
#8977=CARTESIAN_POINT ( 'NONE',  ( 31.00000000000000711, 27.42469319230600533, -6.000000000000006217 ) ) ;
#8979=LINE ( 'NONE', #8284, #9231 ) ;
#8981=VECTOR ( 'NONE', #1755, 1000.000000000000000 ) ;
#8985=CARTESIAN_POINT ( 'NONE',  ( 11.07761026121385939, -5.000000000000008882, 37.39366993089406321 ) ) ;
#8989=DIRECTION ( 'NONE',  ( 0.2840412887490735838, 0.000000000000000000, -0.9588120495101035701 ) ) ;
#8992=CARTESIAN_POINT ( 'NONE',  ( 9.079125748275108876, -7.673965757712833735, 37.92978250830171305 ) ) ;
#8995=ORIENTED_EDGE ( 'NONE', *, *, #7081, .F. ) ;
#8997=ORIENTED_EDGE ( 'NONE', *, *, #3312, .T. ) ;
#9003=CARTESIAN_POINT ( 'NONE',  ( -6.605258697374647880, 10.83052367162449769, 42.87576923823134223 ) ) ;
#9006=B_SPLINE_CURVE_WITH_KNOTS ( 'NONE', 3,
 ( #1505, #1232, #5988, #4248, #6034, #2283, #7950, #7248, #497, #6504, #9526, #2751, #7484, #550 ),
 .UNSPECIFIED., .F., .F.,
 ( 4, 2, 2, 2, 2, 2, 4 ),
 ( 0.01227318291200276898, 0.01534032230130411359, 0.01687389199595478589, 0.01840746169060545820, 0.02147460107990680628, 0.02300817077455747511, 0.02454174046920814395 ),
 .UNSPECIFIED. ) ;
#9008=ORIENTED_EDGE ( 'NONE', *, *, #825, .F. ) ;
#9015=DIRECTION ( 'NONE',  ( -0.000000000000000000, 1.000000000000000000, -0.000000000000000000 ) ) ;
#9019=CARTESIAN_POINT ( 'NONE',  ( -4.007921376381017531, 27.80323177039520388, 31.00000000000000711 ) ) ;
#9026=CARTESIAN_POINT ( 'NONE',  ( 0.1742879017051222057, -14.99999999999999822, 30.58239647876216338 ) ) ;
#9029=CARTESIAN_POINT ( 'NONE',  ( -3.203813853954870616, 17.85736785735978671, 38.86945905611829488 ) ) ;
#9037=DIRECTION ( 'NONE',  ( 1.000000000000000000, 0.000000000000000000, 0.000000000000000000 ) ) ;
#9038=CARTESIAN_POINT ( 'NONE',  ( 10.23892364353549134, -5.543295408803479596, 37.65277200319494000 ) ) ;
#9045=CARTESIAN_POINT ( 'NONE',  ( 11.93007620353410658, 9.934074206894875303, 37.13110854819542794 ) ) ;
#9056=CARTESIAN_POINT ( 'NONE',  ( -6.000000000000005329, 30.00000000000000000, -28.37252191822215863 ) ) ;
#9057=CARTESIAN_POINT ( 'NONE',  ( -10.00000000000001599, 3.294852476658805873, 41.36423575989289247 ) ) ;
#9060=CARTESIAN_POINT ( 'NONE',  ( -6.878531448062598308, -7.640523322561358910, 38.67977308254881308 ) ) ;
#9075=VERTEX_POINT ( 'NONE', #755 ) ;
#9076=DIRECTION ( 'NONE',  ( -1.000000000000000000, 0.000000000000000000, -0.000000000000000000 ) ) ;
#9078=CARTESIAN_POINT ( 'NONE',  ( 7.536700119255284491, -15.00000000000000000, 28.01306679336680006 ) ) ;
#9082=DIRECTION ( 'NONE',  ( -0.000000000000000000, 1.000000000000000000, -0.000000000000000000 ) ) ;
#9085=CIRCLE ( 'NONE', #5761, 39.00000000000002132 ) ;
#9088=DIRECTION ( 'NONE',  ( 0.000000000000000000, 0.000000000000000000, -1.000000000000000000 ) ) ;
#9091=CARTESIAN_POINT ( 'NONE',  ( 7.618647048773172337, -7.203156711660245293, 38.46734435507664074 ) ) ;
#9097=CIRCLE ( 'NONE', #4206, 10.00000000000001599 ) ;
#9100=CARTESIAN_POINT ( 'NONE',  ( 9.655005590677982141, 0.6701487737192702854, 41.54853162078376982 ) ) ;
#9106=CARTESIAN_POINT ( 'NONE',  ( 6.000000000000007994, 29.14236109046821710, 29.24912810952613640 ) ) ;
#9107=ORIENTED_EDGE ( 'NONE', *, *, #868, .F. ) ;
#9114=CARTESIAN_POINT ( 'NONE',  ( -8.670365033978340463, -1.729970272750784410, 42.03780558699289571 ) ) ;
#9119=CARTESIAN_POINT ( 'NONE',  ( -2.303357589342566847, -6.441777582968667204, 43.86679826992887143 ) ) ;
#9121=B_SPLINE_CURVE_WITH_KNOTS ( 'NONE', 3,
 ( #1258, #7976, #4273, #7271 ),
 .UNSPECIFIED., .F., .F.,
 ( 4, 4 ),
 ( 0.000000000000000000, 0.003679109433542032855 ),
 .UNSPECIFIED. ) ;
#9130=CARTESIAN_POINT ( 'NONE',  ( 0.02451486836956002016, 18.29482697815588566, 38.99999229514322252 ) ) ;
#9133=CARTESIAN_POINT ( 'NONE',  ( 26.32489316217636954, -10.00000000000000711, 6.000000000000000000 ) ) ;
#9136=EDGE_LOOP ( 'NONE', ( #9008, #1141, #3358, #9209, #3713, #898, #2959, #9201, #202, #5749, #3053, #2676 ) ) ;
#9137=PLANE ( 'NONE',  #6503 ) ;
#9138=CARTESIAN_POINT ( 'NONE',  ( 2.084579453908214308, -15.00000000000063061, 36.76935723448232096 ) ) ;
#9139=ORIENTED_EDGE ( 'NONE', *, *, #6961, .F. ) ;
#9140=EDGE_CURVE ( 'NONE', #3264, #4918, #357, .T. ) ;
#9142=FACE_OUTER_BOUND ( 'NONE', #8168, .T. ) ;
#9143=CARTESIAN_POINT ( 'NONE',  ( 7.930104434999360130, -2.832236619497283669, 42.36545191093337337 ) ) ;
#9152=CARTESIAN_POINT ( 'NONE',  ( -5.008074634385680568, 27.61318074145110302, -31.00000000000001066 ) ) ;
#9162=ORIENTED_EDGE ( 'NONE', *, *, #4393, .F. ) ;
#9166=CARTESIAN_POINT ( 'NONE',  ( -0.01963426291157483600, -6.705128248126140278, 43.99999014335539016 ) ) ;
#9168=CIRCLE ( 'NONE', #644, 5.000000000000000888 ) ;
#9184=VERTEX_POINT ( 'NONE', #4112 ) ;
#9186=ORIENTED_EDGE ( 'NONE', *, *, #1073, .F. ) ;
#9193=ORIENTED_EDGE ( 'NONE', *, *, #4010, .T. ) ;
#9194=CARTESIAN_POINT ( 'NONE',  ( 4.687036446413768154, -10.75076954218533132, 38.71946050564961439 ) ) ;
#9201=ORIENTED_EDGE ( 'NONE', *, *, #5999, .F. ) ;
#9203=ORIENTED_EDGE ( 'NONE', *, *, #761, .F. ) ;
#9207=LINE ( 'NONE', #8465, #8090 ) ;
#9209=ORIENTED_EDGE ( 'NONE', *, *, #6293, .F. ) ;
#9210=CARTESIAN_POINT ( 'NONE',  ( -3.584397025509258761, -8.971624701663312607, 39.30274302901151628 ) ) ;
#9213=CARTESIAN_POINT ( 'NONE',  ( -4.439212511098975966, -5.714671299323741849, 38.81770112249359528 ) ) ;
#9217=EDGE_CURVE ( 'NONE', #7758, #7231, #8175, .T. ) ;
#9231=VECTOR ( 'NONE', #9666, 1000.000000000000000 ) ;
#9237=VECTOR ( 'NONE', #7521, 1000.000000000000000 ) ;
#9238=CONICAL_SURFACE ( 'NONE', #2588, 10.00000000000001421, 0.07734202994352787353 ) ;
#9254=CARTESIAN_POINT ( 'NONE',  ( -3.582198172489065691, -6.047248247680749422, 43.67305511344584801 ) ) ;
#9257=ORIENTED_EDGE ( 'NONE', *, *, #8799, .T. ) ;
#9261=CARTESIAN_POINT ( 'NONE',  ( -6.118192406390955185, -4.621831477418986367, 43.03401398244064069 ) ) ;
#9262=EDGE_CURVE ( 'NONE', #285, #3751, #2464, .T. ) ;
#9271=ADVANCED_FACE ( 'NONE', ( #600 ), #4216, .T. ) ;
#9276=B_SPLINE_CURVE_WITH_KNOTS ( 'NONE', 3,
 ( #5219, #2182, #5372, #8425, #5424, #8382, #3891, #4637, #8973, #6039, #1614, #5951, #6100, #7592, #8279, #1659, #6884, #3330, #3836, #7441, #8226, #6832, #7489, #5266 ),
 .UNSPECIFIED., .F., .F.,
 ( 4, 2, 2, 2, 2, 2, 2, 2, 2, 2, 2, 4 ),
 ( 0.06349434409688703429, 0.06548129692158807802, 0.06647477333393859988, 0.06746824974628912175, 0.06945520257099015160, 0.07144215539569119533, 0.07342910822039223906, 0.07442258463274276092, 0.07541606104509328279, 0.07640953745744380465, 0.07740301386979431264, 0.07938996669449535637 ),
 .UNSPECIFIED. ) ;
#9287=FACE_OUTER_BOUND ( 'NONE', #8783, .T. ) ;
#9289=CARTESIAN_POINT ( 'NONE',  ( 5.894973159897614501, -10.18605400909195602, 38.56045930014798984 ) ) ;
#9306=CARTESIAN_POINT ( 'NONE',  ( -9.978207696992249964, 4.056654655798920928, 37.86436474176541367 ) ) ;
#9309=ORIENTED_EDGE ( 'NONE', *, *, #7273, .F. ) ;
#9310=DIRECTION ( 'NONE',  ( -1.000000000000000000, 0.000000000000000000, 0.000000000000000000 ) ) ;
#9312=LINE ( 'NONE', #5515, #9681 ) ;
#9315=CARTESIAN_POINT ( 'NONE',  ( 6.000000000000001776, -15.00000000000000000, -31.00000000000000711 ) ) ;
#9325=DIRECTION ( 'NONE',  ( 0.000000000000000000, 0.000000000000000000, 1.000000000000000000 ) ) ;
#9328=EDGE_CURVE ( 'NONE', #7653, #2998, #4790, .T. ) ;
#9331=EDGE_CURVE ( 'NONE', #960, #7928, #5433, .T. ) ;
#9341=VERTEX_POINT ( 'NONE', #6303 ) ;
#9349=VERTEX_POINT ( 'NONE', #7096 ) ;
#9352=CARTESIAN_POINT ( 'NONE',  ( -5.263670707606620702, -5.244400598322866536, 38.72935084317680321 ) ) ;
#9357=ORIENTED_EDGE ( 'NONE', *, *, #6475, .T. ) ;
#9360=CARTESIAN_POINT ( 'NONE',  ( -10.00000000000001421, 3.294852476641298100, 184.6745183374407020 ) ) ;
#9363=CARTESIAN_POINT ( 'NONE',  ( 12.42372165054948141, -2.086834094042897103, 36.96875360800631682 ) ) ;
#9364=DIRECTION ( 'NONE',  ( 0.000000000000000000, -1.000000000000000000, 0.000000000000000000 ) ) ;
#9372=ORIENTED_EDGE ( 'NONE', *, *, #825, .T. ) ;
#9376=CARTESIAN_POINT ( 'NONE',  ( -12.93864508289175141, -0.2176600089833630181, 36.79137408646710838 ) ) ;
#9379=VECTOR ( 'NONE', #6599, 1000.000000000000000 ) ;
#9385=AXIS2_PLACEMENT_3D ( 'NONE', #5758, #4833, #6440 ) ;
#9401=EDGE_LOOP ( 'NONE', ( #2436, #7912, #3553, #3105, #8025 ) ) ;
#9411=CARTESIAN_POINT ( 'NONE',  ( -12.44909004914269168, -1.994056636296514196, 36.96012135774385143 ) ) ;
#9423=DIRECTION ( 'NONE',  ( -0.000000000000000000, 1.000000000000000000, -0.000000000000000000 ) ) ;
#9430=CARTESIAN_POINT ( 'NONE',  ( 0.6802059239249094169, 13.27724345761031799, 43.99097674794369794 ) ) ;
#9438=CARTESIAN_POINT ( 'NONE',  ( 31.00000000000000711, -10.00000000000000533, -6.000000000000006217 ) ) ;
#9441=CARTESIAN_POINT ( 'NONE',  ( -8.825403668520980460, -15.00000000000000000, 36.98508877022077002 ) ) ;
#9448=CARTESIAN_POINT ( 'NONE',  ( 4.458695940319988615, 12.25186834038896677, 43.49095922549461335 ) ) ;
#9456=CARTESIAN_POINT ( 'NONE',  ( -10.82069016047256227, -5.434853743389174596, 37.46967153039774701 ) ) ;
#9467=DIRECTION ( 'NONE',  ( 0.000000000000000000, 0.000000000000000000, 1.000000000000000000 ) ) ;
#9473=CARTESIAN_POINT ( 'NONE',  ( 31.00000000000000711, -10.00000000000000533, 6.000000000000000000 ) ) ;
#9481=VERTEX_POINT ( 'NONE', #7351 ) ;
#9483=CARTESIAN_POINT ( 'NONE',  ( -3.216413334743783103, -15.00000000000062883, 36.77513389234219687 ) ) ;
#9487=CARTESIAN_POINT ( 'NONE',  ( 2.766011525709246577, 12.93636287564932807, 38.93656662069780339 ) ) ;
#9493=ORIENTED_EDGE ( 'NONE', *, *, #7818, .T. ) ;
#9496=CARTESIAN_POINT ( 'NONE',  ( -7.023314015493160589, 16.04054292710173257, 38.36414130246328114 ) ) ;
#9502=CARTESIAN_POINT ( 'NONE',  ( 6.000000000000001776, -10.00000000000000533, -31.00000000000000711 ) ) ;
#9510=CARTESIAN_POINT ( 'NONE',  ( -28.37252191822216218, 30.00000000000000000, -5.999999999999996447 ) ) ;
#9513=EDGE_CURVE ( 'NONE', #9349, #6799, #548, .T. ) ;
#9521=VERTEX_POINT ( 'NONE', #6595 ) ;
#9526=CARTESIAN_POINT ( 'NONE',  ( 9.401064979878146488, -6.093490218539241887, 37.92280751639714254 ) ) ;
#9529=EDGE_LOOP ( 'NONE', ( #968, #3262, #4163, #2085 ) ) ;
#9531=CARTESIAN_POINT ( 'NONE',  ( -0.5763160496995928250, -9.468987443031627649, 39.52686025307730944 ) ) ;
#9538=CARTESIAN_POINT ( 'NONE',  ( 8.174139990748312101, 9.098271002114579176, 38.27377497168703968 ) ) ;
#9552=AXIS2_PLACEMENT_3D ( 'NONE', #6515, #8100, #7364 ) ;
#9559=DIRECTION ( 'NONE',  ( 0.000000000000000000, -1.000000000000000000, 0.000000000000000000 ) ) ;
#9560=CARTESIAN_POINT ( 'NONE',  ( 11.41459187292171151, 11.09818508355548872, 37.29611385600085072 ) ) ;
#9562=EDGE_CURVE ( 'NONE', #9184, #7653, #5326, .T. ) ;
#9565=EDGE_CURVE ( 'NONE', #7120, #6350, #5624, .T. ) ;
#9572=CARTESIAN_POINT ( 'NONE',  ( 9.671127104547153408, 5.921967959015561611, 41.54032951960448372 ) ) ;
#9577=CARTESIAN_POINT ( 'NONE',  ( -12.23816054246644036, -2.710493630309420254, 37.03212527134820675 ) ) ;
#9583=FACE_OUTER_BOUND ( 'NONE', #5061, .T. ) ;
#9586=CARTESIAN_POINT ( 'NONE',  ( -0.1907661894286938054, -15.00000000000000000, 30.58171691558911931 ) ) ;
#9589=DIRECTION ( 'NONE',  ( 0.000000000000000000, 0.000000000000000000, -1.000000000000000000 ) ) ;
#9590=CARTESIAN_POINT ( 'NONE',  ( 7.315962409250510667, 10.12005692215709196, 42.61102608560413785 ) ) ;
#9594=DIRECTION ( 'NONE',  ( -0.000000000000000000, -0.000000000000000000, 1.000000000000000000 ) ) ;
#9598=CARTESIAN_POINT ( 'NONE',  ( -8.358540341008785290, 8.859167319972213406, 38.23848664195695335 ) ) ;
#9601=B_SPLINE_CURVE_WITH_KNOTS ( 'NONE', 3,
 ( #4012, #271, #3260, #2508 ),
 .UNSPECIFIED., .F., .F.,
 ( 4, 4 ),
 ( 0.000000000000000000, 0.003679109433542032855 ),
 .UNSPECIFIED. ) ;
#9602=ORIENTED_EDGE ( 'NONE', *, *, #9217, .T. ) ;
#9613=CARTESIAN_POINT ( 'NONE',  ( 1.342554273002455556, 13.20990960304843931, 43.95670083747006629 ) ) ;
#9619=CARTESIAN_POINT ( 'NONE',  ( -6.000000000000005329, -15.00000000000000000, -26.32489316217636954 ) ) ;
#9624=CARTESIAN_POINT ( 'NONE',  ( -10.67413343474082588, -5.256176925685571710, 37.51319708726573765 ) ) ;
#9629=EDGE_CURVE ( 'NONE', #8756, #1203, #2323, .T. ) ;
#9631=DIRECTION ( 'NONE',  ( -0.000000000000000000, 1.000000000000000000, -0.000000000000000000 ) ) ;
#9632=CARTESIAN_POINT ( 'NONE',  ( 0.8980271448007615120, 18.26880201182753538, 38.99211230656880645 ) ) ;
#9634=AXIS2_PLACEMENT_3D ( 'NONE', #9315, #8577, #3988 ) ;
#9635=VERTEX_POINT ( 'NONE', #779 ) ;
#9642=CARTESIAN_POINT ( 'NONE',  ( -6.647844517998846570, 16.29448827485380136, 38.43121571274925685 ) ) ;
#9654=CARTESIAN_POINT ( 'NONE',  ( 0.000000000000000000, 0.000000000000000000, 0.000000000000000000 ) ) ;
#9664=CARTESIAN_POINT ( 'NONE',  ( 6.848559158202236041, -15.00000000000000178, 28.25275382344465314 ) ) ;
#9666=DIRECTION ( 'NONE',  ( 0.000000000000000000, 0.000000000000000000, 1.000000000000000000 ) ) ;
#9673=CARTESIAN_POINT ( 'NONE',  ( 0.5290539970386457513, -9.461942445008636682, 39.52372684969373040 ) ) ;
#9678=CARTESIAN_POINT ( 'NONE',  ( 12.61936450812443056, 8.119135588597398367, 36.90359936746606451 ) ) ;
#9679=ADVANCED_FACE ( 'NONE', ( #3133 ), #3233, .T. ) ;
#9681=VECTOR ( 'NONE', #328, 1000.000000000000000 ) ;
#9682=ORIENTED_EDGE ( 'NONE', *, *, #1375, .T. ) ;
#9692=CARTESIAN_POINT ( 'NONE',  ( -3.453443797567174123, 17.81395218307918427, 38.85641742718816261 ) ) ;
#9693=CARTESIAN_POINT ( 'NONE',  ( 26.32489316217636954, -15.00000000000000000, -6.000000000000006217 ) ) ;
#9700=DIRECTION ( 'NONE',  ( 0.000000000000000000, 0.000000000000000000, 1.000000000000000000 ) ) ;
#9704=EDGE_CURVE ( 'NONE', #8597, #7666, #7389, .T. ) ;
#9721=CARTESIAN_POINT ( 'NONE',  ( 29.24912810952613640, 29.14236109046821710, -6.000000000000006217 ) ) ;
#9722=CARTESIAN_POINT ( 'NONE',  ( -6.150308060456896264, 16.61224636055649384, 38.51628361999085115 ) ) ;
#9723=ADVANCED_FACE ( 'NONE', ( #4329 ), #5019, .T. ) ;
#9728=CARTESIAN_POINT ( 'NONE',  ( 11.07761026121385584, -15.00000000000000000, 37.39366993089404900 ) ) ;
#9730=CARTESIAN_POINT ( 'NONE',  ( 0.000000000000000000, -15.00000000000000000, 0.000000000000000000 ) ) ;
#9734=CARTESIAN_POINT ( 'NONE',  ( 7.039660980758952746, -3.873581541912419546, 38.48359011748724612 ) ) ;
#9743=CARTESIAN_POINT ( 'NONE',  ( -4.444672669478428872, 12.25879546470133974, 43.49417769924191646 ) ) ;
#9744=EDGE_CURVE ( 'NONE', #874, #1345, #8817, .T. ) ;
#9745=DIRECTION ( 'NONE',  ( 0.000000000000000000, 0.000000000000000000, -1.000000000000000000 ) ) ;
#9747=DIRECTION ( 'NONE',  ( 0.000000000000000000, 0.000000000000000000, -1.000000000000000000 ) ) ;
#9748=ADVANCED_BREP_SHAPE_REPRESENTATION ( '', ( #6323, #6314 ), #2196 ) ;
#9750=CARTESIAN_POINT ( 'NONE',  ( -7.740900945811527656, -7.145159734021766518, 38.44003917021594674 ) ) ;
#9751=CARTESIAN_POINT ( 'NONE',  ( 6.000000000000001776, 27.42469319230600533, -31.00000000000000711 ) ) ;
#9765=COLOUR_RGB('Dark Blue',0.08,0.2,0.34);
#9766=FILL_AREA_STYLE_COLOUR('',#9765);
#9767=FILL_AREA_STYLE('',(#9766));
#9768=SURFACE_STYLE_FILL_AREA(#9767);
#9769=SURFACE_SIDE_STYLE('',(#9768));
#9770=SURFACE_STYLE_USAGE(.BOTH.,#9769);
#9771=PRESENTATION_STYLE_ASSIGNMENT((#9770));
ENDSEC;
END-ISO-10303-21;
